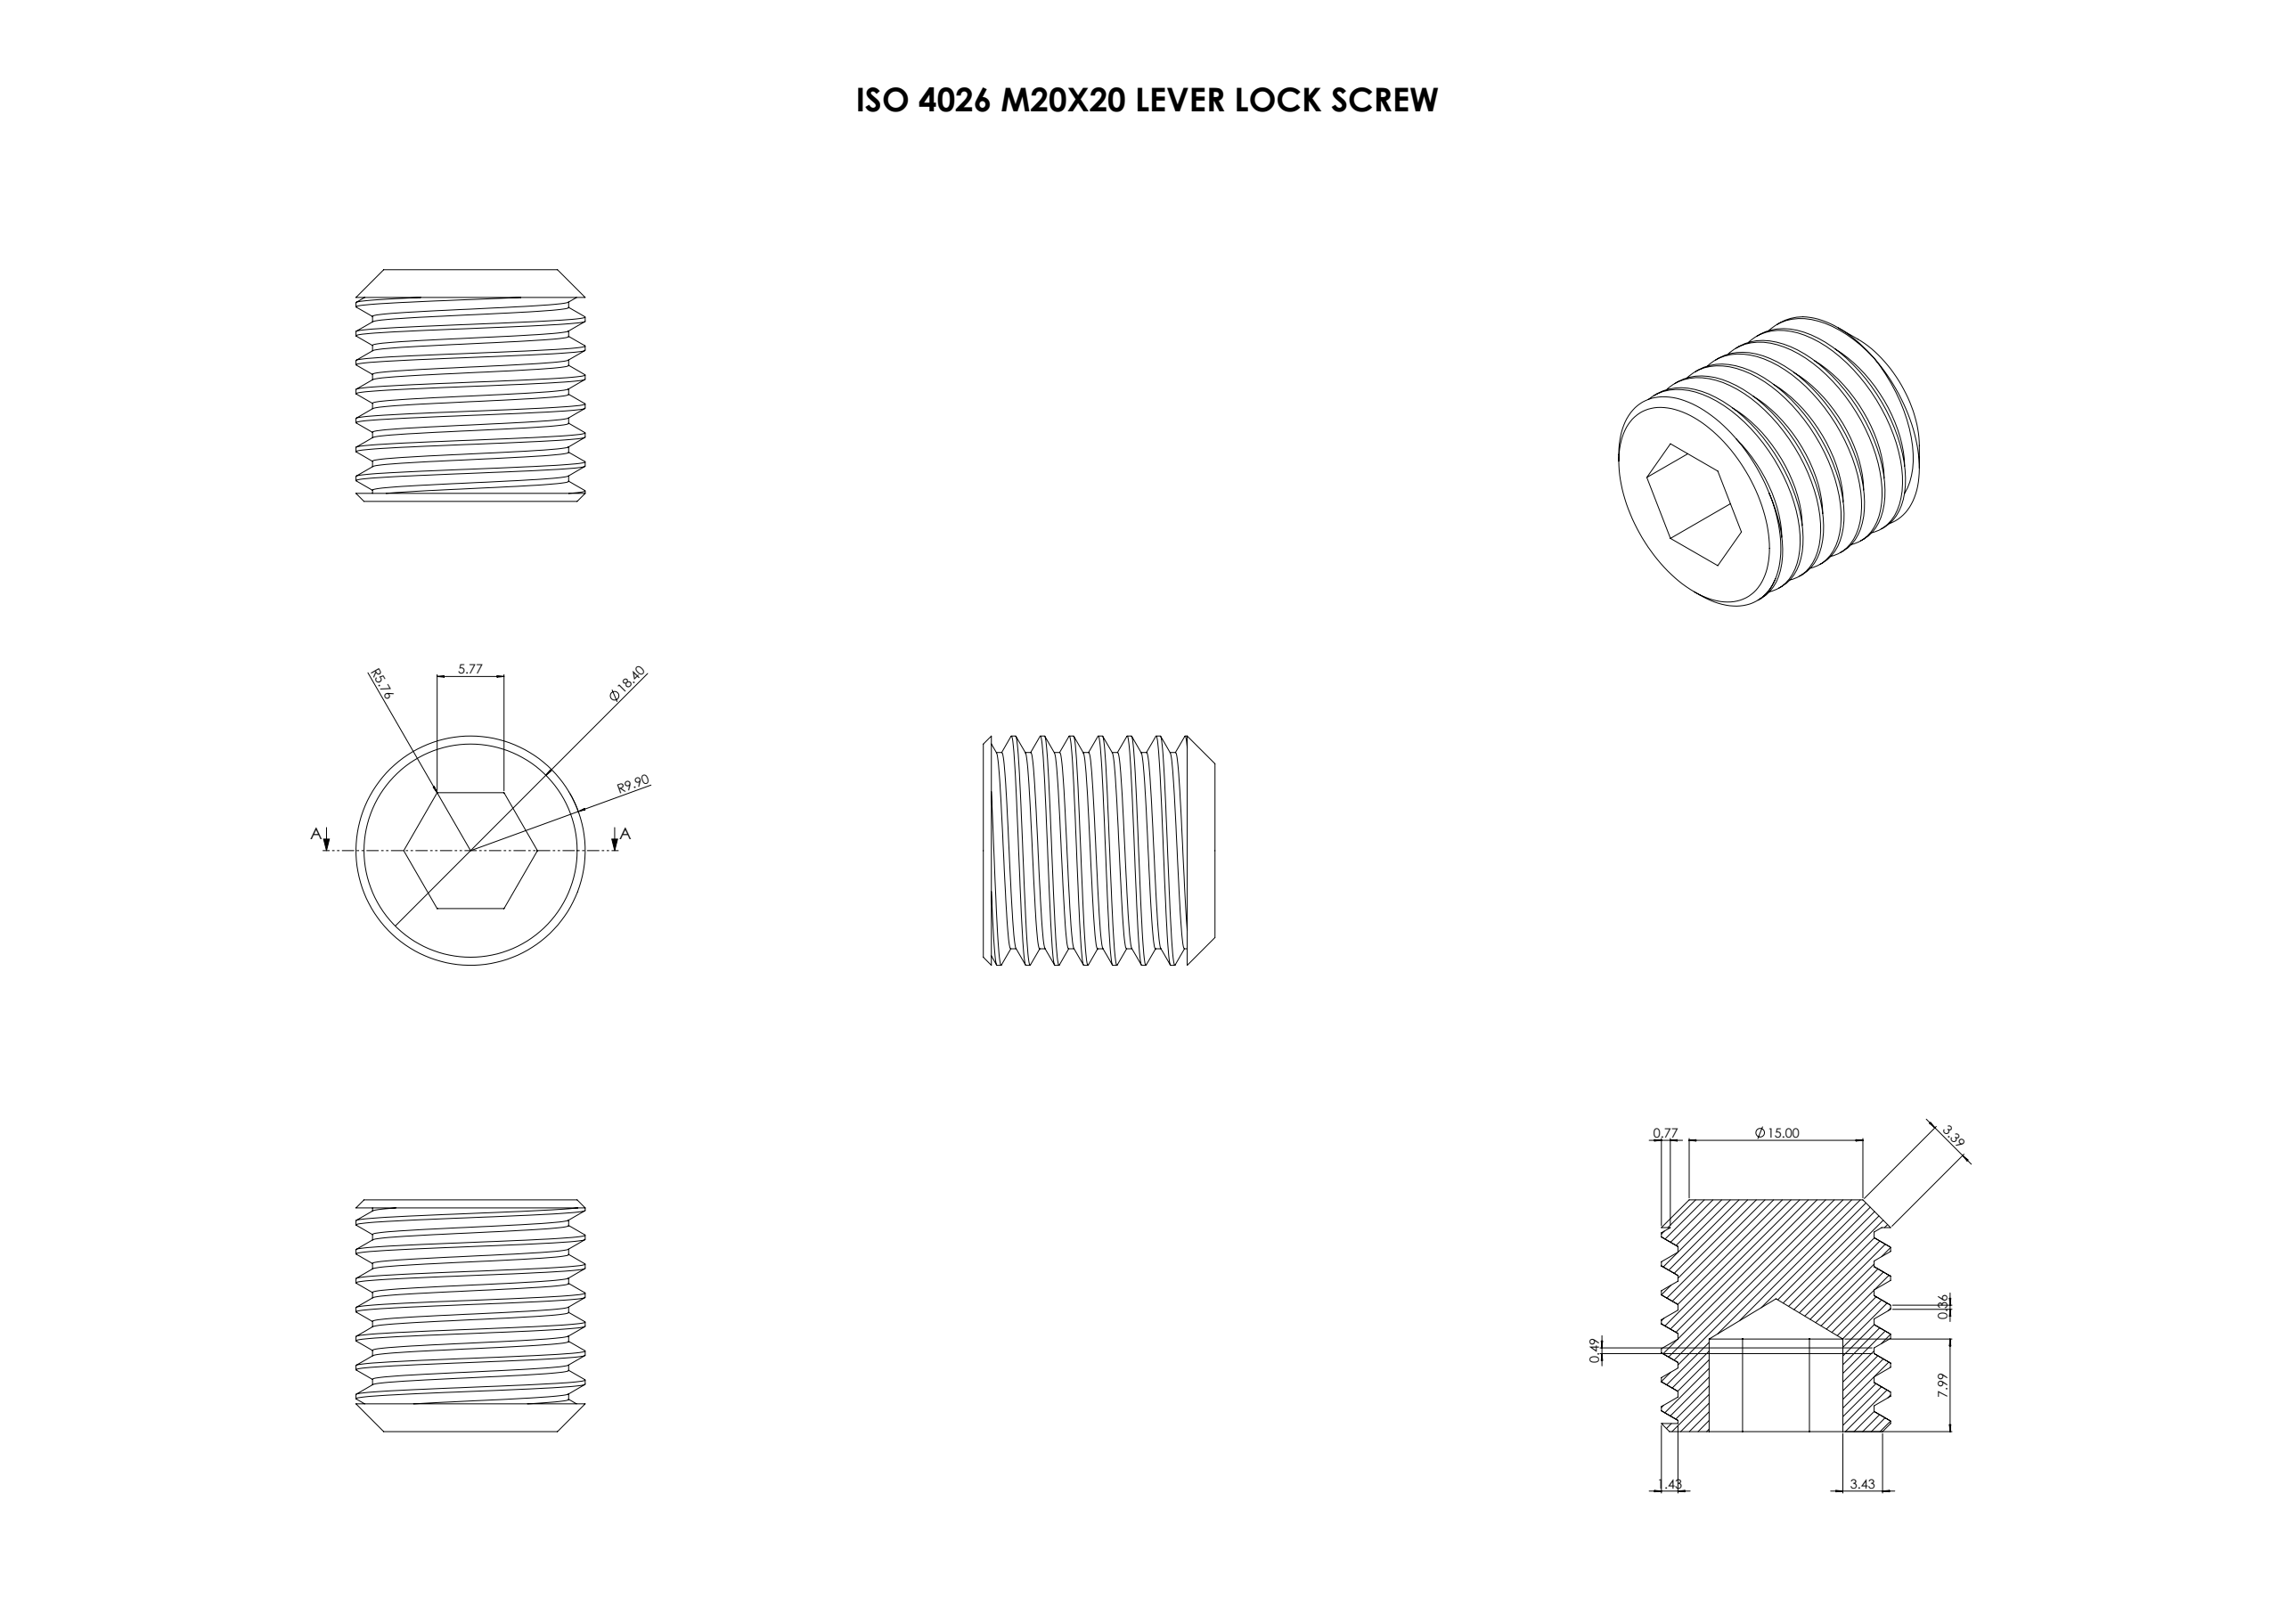
ISO-10303-21;
HEADER;
/* Generated by software containing ST-Developer
 * from STEP Tools, Inc. (www.steptools.com) 
 */

FILE_DESCRIPTION(
/* description */ (''),
/* implementation_level */ '2;1');

FILE_NAME(
/* name */ '15_ISO_4026_M20x20_Lever_Lock_Screw.step',
/* time_stamp */ '2026-10-19T23:58:09-07:00',
/* author */ (''),
/* organization */ (''),
/* preprocessor_version */ 'ST-DEVELOPER v20.2',
/* originating_system */ 'Autodesk Translation Framework v15.15.0.0',
/* authorisation */ '');

FILE_SCHEMA (('AP203_CONFIGURATION_CONTROLLED_3D_DESIGN_OF_MECHANICAL_PARTS_AND_ASSEMBLIES_MIM_LF { 1 0 10303 203 3 1 4 }',
'AUTOMOTIVE_DESIGN { 1 0 10303 214 3 1 1 }','INTEGRATED_CNC_SCHEMA','MODEL_BASED_INTEGRATED_MANUFACTURING_SCHEMA',
'PROCESS_PLANNING_SCHEMA','AP242_MANAGED_MODEL_BASED_3D_ENGINEERING_MIM_LF { 1 0 10303 442 3 1 4 }'));
ENDSEC;

DATA;
#10=MECHANICAL_DESIGN_GEOMETRIC_PRESENTATION_REPRESENTATION('',(#412),#70757);
#203=(
BOUNDED_CURVE()
B_SPLINE_CURVE(2,(#47308,#47309,#47310),.UNSPECIFIED.,.F.,.F.)
B_SPLINE_CURVE_WITH_KNOTS((3,3),(0.,0.00348481894602421),.UNSPECIFIED.)
CURVE()
GEOMETRIC_REPRESENTATION_ITEM()
RATIONAL_B_SPLINE_CURVE((1.,1.00000419109631,1.))
REPRESENTATION_ITEM('')
);
#204=(
BOUNDED_CURVE()
B_SPLINE_CURVE(2,(#47312,#47313,#47314),.UNSPECIFIED.,.F.,.F.)
B_SPLINE_CURVE_WITH_KNOTS((3,3),(0.,0.0034848189460241),.UNSPECIFIED.)
CURVE()
GEOMETRIC_REPRESENTATION_ITEM()
RATIONAL_B_SPLINE_CURVE((1.,1.00000419078036,1.))
REPRESENTATION_ITEM('')
);
#205=(
BOUNDED_CURVE()
B_SPLINE_CURVE(2,(#47317,#47318,#47319),.UNSPECIFIED.,.F.,.F.)
B_SPLINE_CURVE_WITH_KNOTS((3,3),(0.,0.00348481894602397),.UNSPECIFIED.)
CURVE()
GEOMETRIC_REPRESENTATION_ITEM()
RATIONAL_B_SPLINE_CURVE((1.,1.00000419109938,1.))
REPRESENTATION_ITEM('')
);
#206=(
BOUNDED_CURVE()
B_SPLINE_CURVE(2,(#47321,#47322,#47323),.UNSPECIFIED.,.F.,.F.)
B_SPLINE_CURVE_WITH_KNOTS((3,3),(0.,0.00348481894602389),.UNSPECIFIED.)
CURVE()
GEOMETRIC_REPRESENTATION_ITEM()
RATIONAL_B_SPLINE_CURVE((1.,1.0000041910806,1.))
REPRESENTATION_ITEM('')
);
#207=(
BOUNDED_CURVE()
B_SPLINE_CURVE(2,(#47326,#47327,#47328),.UNSPECIFIED.,.F.,.F.)
B_SPLINE_CURVE_WITH_KNOTS((3,3),(0.,0.003484818946024),.UNSPECIFIED.)
CURVE()
GEOMETRIC_REPRESENTATION_ITEM()
RATIONAL_B_SPLINE_CURVE((1.,1.00000419096159,1.))
REPRESENTATION_ITEM('')
);
#208=(
BOUNDED_CURVE()
B_SPLINE_CURVE(2,(#47330,#47331,#47332),.UNSPECIFIED.,.F.,.F.)
B_SPLINE_CURVE_WITH_KNOTS((3,3),(0.,0.00348481894602396),.UNSPECIFIED.)
CURVE()
GEOMETRIC_REPRESENTATION_ITEM()
RATIONAL_B_SPLINE_CURVE((1.,1.00000419112827,1.))
REPRESENTATION_ITEM('')
);
#209=(
BOUNDED_CURVE()
B_SPLINE_CURVE(2,(#47335,#47336,#47337),.UNSPECIFIED.,.F.,.F.)
B_SPLINE_CURVE_WITH_KNOTS((3,3),(0.,0.00348481894602387),.UNSPECIFIED.)
CURVE()
GEOMETRIC_REPRESENTATION_ITEM()
RATIONAL_B_SPLINE_CURVE((1.,1.00000419105483,1.))
REPRESENTATION_ITEM('')
);
#210=(
BOUNDED_CURVE()
B_SPLINE_CURVE(2,(#47339,#47340,#47341),.UNSPECIFIED.,.F.,.F.)
B_SPLINE_CURVE_WITH_KNOTS((3,3),(0.,0.00348481894602378),.UNSPECIFIED.)
CURVE()
GEOMETRIC_REPRESENTATION_ITEM()
RATIONAL_B_SPLINE_CURVE((1.,1.00000419099658,1.))
REPRESENTATION_ITEM('')
);
#211=(
BOUNDED_CURVE()
B_SPLINE_CURVE(2,(#47344,#47345,#47346),.UNSPECIFIED.,.F.,.F.)
B_SPLINE_CURVE_WITH_KNOTS((3,3),(0.,0.00348481894602419),.UNSPECIFIED.)
CURVE()
GEOMETRIC_REPRESENTATION_ITEM()
RATIONAL_B_SPLINE_CURVE((1.,1.00000419117121,1.))
REPRESENTATION_ITEM('')
);
#212=(
BOUNDED_CURVE()
B_SPLINE_CURVE(2,(#47348,#47349,#47350),.UNSPECIFIED.,.F.,.F.)
B_SPLINE_CURVE_WITH_KNOTS((3,3),(0.,0.00348481894602411),.UNSPECIFIED.)
CURVE()
GEOMETRIC_REPRESENTATION_ITEM()
RATIONAL_B_SPLINE_CURVE((1.,1.00000419088834,1.))
REPRESENTATION_ITEM('')
);
#213=(
BOUNDED_CURVE()
B_SPLINE_CURVE(2,(#47353,#47354,#47355),.UNSPECIFIED.,.F.,.F.)
B_SPLINE_CURVE_WITH_KNOTS((3,3),(0.,0.00348481894602378),.UNSPECIFIED.)
CURVE()
GEOMETRIC_REPRESENTATION_ITEM()
RATIONAL_B_SPLINE_CURVE((1.,1.00000419109063,1.))
REPRESENTATION_ITEM('')
);
#214=(
BOUNDED_CURVE()
B_SPLINE_CURVE(2,(#47357,#47358,#47359),.UNSPECIFIED.,.F.,.F.)
B_SPLINE_CURVE_WITH_KNOTS((3,3),(0.,0.00348481894602365),.UNSPECIFIED.)
CURVE()
GEOMETRIC_REPRESENTATION_ITEM()
RATIONAL_B_SPLINE_CURVE((1.,1.00000419111732,1.))
REPRESENTATION_ITEM('')
);
#274=B_SPLINE_SURFACE_WITH_KNOTS('',3,3,((#46301,#46302,#46303,#46304,#46305,
#46306,#46307,#46308,#46309,#46310,#46311,#46312,#46313,#46314,#46315,#46316,
#46317,#46318,#46319,#46320,#46321,#46322,#46323,#46324,#46325,#46326,#46327,
#46328,#46329,#46330,#46331,#46332,#46333,#46334,#46335,#46336,#46337,#46338,
#46339,#46340,#46341,#46342,#46343,#46344,#46345,#46346,#46347,#46348,#46349,
#46350,#46351,#46352,#46353,#46354,#46355,#46356,#46357,#46358,#46359,#46360,
#46361,#46362,#46363,#46364,#46365,#46366,#46367,#46368,#46369,#46370,#46371,
#46372,#46373,#46374,#46375,#46376,#46377,#46378,#46379,#46380,#46381,#46382,
#46383,#46384,#46385,#46386,#46387,#46388,#46389,#46390,#46391,#46392,#46393),
(#46394,#46395,#46396,#46397,#46398,#46399,#46400,#46401,#46402,#46403,
#46404,#46405,#46406,#46407,#46408,#46409,#46410,#46411,#46412,#46413,#46414,
#46415,#46416,#46417,#46418,#46419,#46420,#46421,#46422,#46423,#46424,#46425,
#46426,#46427,#46428,#46429,#46430,#46431,#46432,#46433,#46434,#46435,#46436,
#46437,#46438,#46439,#46440,#46441,#46442,#46443,#46444,#46445,#46446,#46447,
#46448,#46449,#46450,#46451,#46452,#46453,#46454,#46455,#46456,#46457,#46458,
#46459,#46460,#46461,#46462,#46463,#46464,#46465,#46466,#46467,#46468,#46469,
#46470,#46471,#46472,#46473,#46474,#46475,#46476,#46477,#46478,#46479,#46480,
#46481,#46482,#46483,#46484,#46485,#46486),(#46487,#46488,#46489,#46490,
#46491,#46492,#46493,#46494,#46495,#46496,#46497,#46498,#46499,#46500,#46501,
#46502,#46503,#46504,#46505,#46506,#46507,#46508,#46509,#46510,#46511,#46512,
#46513,#46514,#46515,#46516,#46517,#46518,#46519,#46520,#46521,#46522,#46523,
#46524,#46525,#46526,#46527,#46528,#46529,#46530,#46531,#46532,#46533,#46534,
#46535,#46536,#46537,#46538,#46539,#46540,#46541,#46542,#46543,#46544,#46545,
#46546,#46547,#46548,#46549,#46550,#46551,#46552,#46553,#46554,#46555,#46556,
#46557,#46558,#46559,#46560,#46561,#46562,#46563,#46564,#46565,#46566,#46567,
#46568,#46569,#46570,#46571,#46572,#46573,#46574,#46575,#46576,#46577,#46578,
#46579),(#46580,#46581,#46582,#46583,#46584,#46585,#46586,#46587,#46588,
#46589,#46590,#46591,#46592,#46593,#46594,#46595,#46596,#46597,#46598,#46599,
#46600,#46601,#46602,#46603,#46604,#46605,#46606,#46607,#46608,#46609,#46610,
#46611,#46612,#46613,#46614,#46615,#46616,#46617,#46618,#46619,#46620,#46621,
#46622,#46623,#46624,#46625,#46626,#46627,#46628,#46629,#46630,#46631,#46632,
#46633,#46634,#46635,#46636,#46637,#46638,#46639,#46640,#46641,#46642,#46643,
#46644,#46645,#46646,#46647,#46648,#46649,#46650,#46651,#46652,#46653,#46654,
#46655,#46656,#46657,#46658,#46659,#46660,#46661,#46662,#46663,#46664,#46665,
#46666,#46667,#46668,#46669,#46670,#46671,#46672)),.UNSPECIFIED.,.F.,.F.,
 .F.,(4,4),(4,1,1,1,1,1,1,1,1,1,1,1,1,1,1,1,1,1,1,1,1,1,1,1,1,1,1,1,1,1,
1,1,1,1,1,1,1,1,1,1,1,1,1,1,1,1,1,1,1,1,1,1,1,1,1,1,1,1,1,1,1,1,1,1,1,1,
1,1,1,1,1,1,1,1,1,1,1,1,1,1,1,1,1,1,1,1,1,1,1,1,4),(0.,0.164689164286341),
(8.30638927278254,8.80158653784135,9.29678380290015,9.79198106795896,10.2871783330178,
10.7823755980766,11.2775728631354,11.7727701281942,12.267967393253,12.7631646583118,
13.2583619233706,13.7535591884294,14.2487564534882,14.743953718547,15.2391509836058,
15.7343482486646,16.2295455137234,16.7247427787822,17.219940043841,17.7151373088998,
18.2103345739587,18.7055318390175,19.2007291040763,19.6959263691351,20.1911236341939,
20.6863208992527,21.1815181643115,21.6767154293703,22.1719126944291,22.6671099594879,
23.1623072245467,23.6575044896055,24.1527017546643,24.6478990197231,25.1430962847819,
25.6382935498407,26.1334908148995,26.6286880799584,27.1238853450172,27.619082610076,
28.1142798751348,28.6094771401936,29.1046744052524,29.5998716703112,30.09506893537,
30.5902662004288,31.0854634654876,31.5806607305464,32.0758579956052,32.571055260664,
33.0662525257228,33.5614497907816,34.0566470558404,34.5518443208992,35.0470415859581,
35.5422388510169,36.0374361160757,36.5326333811345,37.0278306461933,37.5230279112521,
38.0182251763109,38.5134224413697,39.0086197064285,39.5038169714873,39.9990142365461,
40.4942115016049,40.9894087666637,41.4846060317225,41.9798032967813,42.4750005618401,
42.9701978268989,43.4653950919578,43.9605923570166,44.4557896220754,44.9509868871342,
45.446184152193,45.9413814172518,46.4365786823106,46.9317759473694,47.4269732124282,
47.922170477487,48.4173677425458,48.9125650076046,49.4077622726634,49.9029595377222,
50.398156802781,50.8933540678398,51.3885513328986,51.8837485979574,52.3789458630163,
52.8741431280751),.UNSPECIFIED.);
#275=B_SPLINE_SURFACE_WITH_KNOTS('',3,3,((#46887,#46888,#46889,#46890,#46891,
#46892,#46893,#46894,#46895,#46896,#46897,#46898,#46899,#46900,#46901,#46902,
#46903,#46904,#46905,#46906,#46907,#46908,#46909,#46910,#46911,#46912,#46913,
#46914,#46915,#46916,#46917,#46918,#46919,#46920,#46921,#46922,#46923,#46924,
#46925,#46926,#46927,#46928,#46929,#46930,#46931,#46932,#46933,#46934,#46935,
#46936,#46937,#46938,#46939,#46940,#46941,#46942,#46943,#46944,#46945,#46946,
#46947,#46948,#46949,#46950,#46951,#46952,#46953,#46954,#46955,#46956,#46957,
#46958,#46959,#46960,#46961,#46962,#46963,#46964,#46965,#46966,#46967,#46968,
#46969,#46970,#46971,#46972,#46973,#46974,#46975,#46976,#46977,#46978,#46979),
(#46980,#46981,#46982,#46983,#46984,#46985,#46986,#46987,#46988,#46989,
#46990,#46991,#46992,#46993,#46994,#46995,#46996,#46997,#46998,#46999,#47000,
#47001,#47002,#47003,#47004,#47005,#47006,#47007,#47008,#47009,#47010,#47011,
#47012,#47013,#47014,#47015,#47016,#47017,#47018,#47019,#47020,#47021,#47022,
#47023,#47024,#47025,#47026,#47027,#47028,#47029,#47030,#47031,#47032,#47033,
#47034,#47035,#47036,#47037,#47038,#47039,#47040,#47041,#47042,#47043,#47044,
#47045,#47046,#47047,#47048,#47049,#47050,#47051,#47052,#47053,#47054,#47055,
#47056,#47057,#47058,#47059,#47060,#47061,#47062,#47063,#47064,#47065,#47066,
#47067,#47068,#47069,#47070,#47071,#47072),(#47073,#47074,#47075,#47076,
#47077,#47078,#47079,#47080,#47081,#47082,#47083,#47084,#47085,#47086,#47087,
#47088,#47089,#47090,#47091,#47092,#47093,#47094,#47095,#47096,#47097,#47098,
#47099,#47100,#47101,#47102,#47103,#47104,#47105,#47106,#47107,#47108,#47109,
#47110,#47111,#47112,#47113,#47114,#47115,#47116,#47117,#47118,#47119,#47120,
#47121,#47122,#47123,#47124,#47125,#47126,#47127,#47128,#47129,#47130,#47131,
#47132,#47133,#47134,#47135,#47136,#47137,#47138,#47139,#47140,#47141,#47142,
#47143,#47144,#47145,#47146,#47147,#47148,#47149,#47150,#47151,#47152,#47153,
#47154,#47155,#47156,#47157,#47158,#47159,#47160,#47161,#47162,#47163,#47164,
#47165),(#47166,#47167,#47168,#47169,#47170,#47171,#47172,#47173,#47174,
#47175,#47176,#47177,#47178,#47179,#47180,#47181,#47182,#47183,#47184,#47185,
#47186,#47187,#47188,#47189,#47190,#47191,#47192,#47193,#47194,#47195,#47196,
#47197,#47198,#47199,#47200,#47201,#47202,#47203,#47204,#47205,#47206,#47207,
#47208,#47209,#47210,#47211,#47212,#47213,#47214,#47215,#47216,#47217,#47218,
#47219,#47220,#47221,#47222,#47223,#47224,#47225,#47226,#47227,#47228,#47229,
#47230,#47231,#47232,#47233,#47234,#47235,#47236,#47237,#47238,#47239,#47240,
#47241,#47242,#47243,#47244,#47245,#47246,#47247,#47248,#47249,#47250,#47251,
#47252,#47253,#47254,#47255,#47256,#47257,#47258)),.UNSPECIFIED.,.F.,.F.,
 .F.,(4,4),(4,1,1,1,1,1,1,1,1,1,1,1,1,1,1,1,1,1,1,1,1,1,1,1,1,1,1,1,1,1,
1,1,1,1,1,1,1,1,1,1,1,1,1,1,1,1,1,1,1,1,1,1,1,1,1,1,1,1,1,1,1,1,1,1,1,1,
1,1,1,1,1,1,1,1,1,1,1,1,1,1,1,1,1,1,1,1,1,1,1,1,4),(0.,0.164689164286341),
(11.6152142277547,12.1104114928135,12.6056087578723,13.1008060229311,13.59600328799,
14.0912005530488,14.5863978181076,15.0815950831664,15.5767923482252,16.071989613284,
16.5671868783428,17.0623841434016,17.5575814084604,18.0527786735192,18.547975938578,
19.0431732036368,19.5383704686956,20.0335677337544,20.5287649988132,21.023962263872,
21.5191595289308,22.0143567939897,22.5095540590485,23.0047513241073,23.4999485891661,
23.9951458542249,24.4903431192837,24.9855403843425,25.4807376494013,25.9759349144601,
26.4711321795189,26.9663294445777,27.4615267096365,27.9567239746953,28.4519212397541,
28.9471185048129,29.4423157698717,29.9375130349305,30.4327102999894,30.9279075650482,
31.423104830107,31.9183020951658,32.4134993602246,32.9086966252834,33.4038938903422,
33.899091155401,34.3942884204598,34.8894856855186,35.3846829505774,35.8798802156362,
36.375077480695,36.8702747457538,37.3654720108126,37.8606692758714,38.3558665409303,
38.8510638059891,39.3462610710479,39.8414583361067,40.3366556011655,40.8318528662243,
41.3270501312831,41.8222473963419,42.3174446614007,42.8126419264595,43.3078391915183,
43.8030364565771,44.2982337216359,44.7934309866947,45.2886282517535,45.7838255168123,
46.2790227818711,46.7742200469299,47.2694173119888,47.7646145770476,48.2598118421064,
48.7550091071652,49.250206372224,49.7454036372828,50.2406009023416,50.7357981674004,
51.2309954324592,51.726192697518,52.2213899625768,52.7165872276356,53.2117844926944,
53.7069817577532,54.202179022812,54.6973762878708,55.1925735529296,55.6877708179885,
56.1829680830473),.UNSPECIFIED.);
#382=SHAPE_REPRESENTATION_RELATIONSHIP('SRR','None',#70823,#397);
#397=ADVANCED_BREP_SHAPE_REPRESENTATION('',(#472),#70747);
#412=STYLED_ITEM('',(#71054),#472);
#472=MANIFOLD_SOLID_BREP('Set screw',#26877);
#606=CYLINDRICAL_SURFACE('',#27433,0.989525);
#607=CYLINDRICAL_SURFACE('',#27435,0.989525);
#608=CYLINDRICAL_SURFACE('',#27436,0.989525);
#609=CYLINDRICAL_SURFACE('',#27437,0.989525);
#610=CYLINDRICAL_SURFACE('',#27438,0.989525);
#611=CYLINDRICAL_SURFACE('',#27439,0.989525);
#612=CYLINDRICAL_SURFACE('',#27440,0.989525);
#613=CYLINDRICAL_SURFACE('',#27441,0.8469);
#614=CYLINDRICAL_SURFACE('',#27443,0.8469);
#615=CYLINDRICAL_SURFACE('',#27445,0.8469);
#616=CYLINDRICAL_SURFACE('',#27446,0.8469);
#617=CYLINDRICAL_SURFACE('',#27447,0.8469);
#618=CYLINDRICAL_SURFACE('',#27448,0.8469);
#619=CYLINDRICAL_SURFACE('',#27449,0.8469);
#620=CYLINDRICAL_SURFACE('',#27457,0.8469);
#621=CYLINDRICAL_SURFACE('',#27505,0.989525);
#861=FACE_BOUND('',#4381,.T.);
#1135=B_SPLINE_CURVE_WITH_KNOTS('',3,(#45348,#45349,#45350,#45351,#45352,
#45353,#45354,#45355,#45356,#45357,#45358,#45359,#45360,#45361,#45362,#45363),
 .UNSPECIFIED.,.F.,.F.,(4,3,3,3,3,4),(-4.09274904019422,-3.96157812047045,
-3.46638085541164,-2.97118359035283,-2.47598632529403,-2.06954507459125),
 .UNSPECIFIED.);
#1136=B_SPLINE_CURVE_WITH_KNOTS('',3,(#45366,#45367,#45368,#45369,#45370,
#45371,#45372,#45373,#45374,#45375),.UNSPECIFIED.,.F.,.F.,(4,3,3,4),(0.,
0.495197265058804,0.990394530117612,1.11838868798682),.UNSPECIFIED.);
#1137=B_SPLINE_CURVE_WITH_KNOTS('',3,(#45380,#45381,#45382,#45383,#45384,
#45385,#45386,#45387,#45388,#45389,#45390,#45391,#45392,#45393,#45394,#45395,
#45396,#45397,#45398,#45399,#45400,#45401,#45402,#45403,#45404,#45405,#45406,
#45407,#45408,#45409,#45410,#45411,#45412,#45413,#45414,#45415,#45416,#45417,
#45418,#45419),.UNSPECIFIED.,.F.,.F.,(4,3,3,3,3,3,3,3,3,3,3,3,3,4),(-10.3759343473738,
-9.90394530117612,-9.40874803611731,-8.91355077105851,-8.4183535059997,
-7.9231562409409,-7.42795897588209,-6.93276171082328,-6.43756444576448,
-5.94236718070567,-5.44716991564687,-4.95197265058806,-4.45677538552925,
-4.09274904019422),.UNSPECIFIED.);
#1138=B_SPLINE_CURVE_WITH_KNOTS('',3,(#45420,#45421,#45422,#45423,#45424,
#45425,#45426,#45427,#45428,#45429,#45430,#45431,#45432,#45433,#45434,#45435,
#45436,#45437,#45438,#45439,#45440,#45441,#45442,#45443,#45444,#45445,#45446,
#45447,#45448,#45449,#45450,#45451,#45452,#45453,#45454,#45455,#45456,#45457,
#45458,#45459),.UNSPECIFIED.,.F.,.F.,(4,3,3,3,3,3,3,3,3,3,3,3,3,4),(1.11838868798682,
1.48559179517642,1.98078906023522,2.47598632529403,2.97118359035284,3.46638085541164,
3.96157812047045,4.45677538552925,4.95197265058806,5.44716991564687,5.94236718070567,
6.43756444576448,6.93276171082328,7.4015739951664),.UNSPECIFIED.);
#1139=B_SPLINE_CURVE_WITH_KNOTS('',3,(#45464,#45465,#45466,#45467,#45468,
#45469,#45470,#45471,#45472,#45473,#45474,#45475,#45476,#45477,#45478,#45479,
#45480,#45481,#45482,#45483,#45484,#45485,#45486,#45487,#45488,#45489,#45490,
#45491,#45492,#45493,#45494,#45495,#45496,#45497,#45498,#45499,#45500,#45501,
#45502,#45503,#45504,#45505,#45506),.UNSPECIFIED.,.F.,.F.,(4,3,3,3,3,3,
3,3,3,3,3,3,3,3,4),(-16.6591196545534,-16.3415097469406,-15.8463124818818,
-15.351115216823,-14.8559179517642,-14.3607206867054,-13.8655234216466,
-13.3703261565878,-12.875128891529,-12.3799316264701,-11.8847343614113,
-11.3895370963525,-10.8943398312937,-10.3991425662349,-10.3759343473738),
 .UNSPECIFIED.);
#1140=B_SPLINE_CURVE_WITH_KNOTS('',3,(#45507,#45508,#45509,#45510,#45511,
#45512,#45513,#45514,#45515,#45516,#45517,#45518,#45519,#45520,#45521,#45522,
#45523,#45524,#45525,#45526,#45527,#45528,#45529,#45530,#45531,#45532,#45533,
#45534,#45535,#45536,#45537,#45538,#45539,#45540,#45541,#45542,#45543,#45544,
#45545,#45546,#45547,#45548,#45549),.UNSPECIFIED.,.F.,.F.,(4,3,3,3,3,3,
3,3,3,3,3,3,3,3,4),(7.4015739951664,7.42795897588209,7.92315624094089,8.4183535059997,
8.9135507710585,9.40874803611731,9.90394530117612,10.3991425662349,10.8943398312937,
11.3895370963525,11.8847343614113,12.3799316264701,12.875128891529,13.3703261565878,
13.684759302346),.UNSPECIFIED.);
#1141=B_SPLINE_CURVE_WITH_KNOTS('',3,(#45554,#45555,#45556,#45557,#45558,
#45559,#45560,#45561,#45562,#45563,#45564,#45565,#45566,#45567,#45568,#45569,
#45570,#45571,#45572,#45573,#45574,#45575,#45576,#45577,#45578,#45579,#45580,
#45581,#45582,#45583,#45584,#45585,#45586,#45587,#45588,#45589,#45590,#45591,
#45592,#45593,#45594,#45595,#45596),.UNSPECIFIED.,.F.,.F.,(4,3,3,3,3,3,
3,3,3,3,3,3,3,3,4),(-22.942304961733,-22.7790741927051,-22.2838769276463,
-21.7886796625875,-21.2934823975287,-20.7982851324699,-20.303087867411,
-19.8078906023522,-19.3126933372934,-18.8174960722346,-18.3222988071758,
-17.827101542117,-17.3319042770582,-16.8367070119994,-16.6591196545534),
 .UNSPECIFIED.);
#1142=B_SPLINE_CURVE_WITH_KNOTS('',3,(#45597,#45598,#45599,#45600,#45601,
#45602,#45603,#45604,#45605,#45606,#45607,#45608,#45609,#45610,#45611,#45612,
#45613,#45614,#45615,#45616,#45617,#45618,#45619,#45620,#45621,#45622,#45623,
#45624,#45625,#45626,#45627,#45628,#45629,#45630,#45631,#45632,#45633,#45634,
#45635,#45636,#45637,#45638,#45639),.UNSPECIFIED.,.F.,.F.,(4,3,3,3,3,3,
3,3,3,3,3,3,3,3,4),(13.684759302346,13.8655234216466,14.3607206867054,14.8559179517642,
15.351115216823,15.8463124818818,16.3415097469406,16.8367070119994,17.3319042770582,
17.827101542117,18.3222988071758,18.8174960722346,19.3126933372934,19.8078906023522,
19.9679446095256),.UNSPECIFIED.);
#1143=B_SPLINE_CURVE_WITH_KNOTS('',3,(#45644,#45645,#45646,#45647,#45648,
#45649,#45650,#45651,#45652,#45653,#45654,#45655,#45656,#45657,#45658,#45659,
#45660,#45661,#45662,#45663,#45664,#45665,#45666,#45667,#45668,#45669,#45670,
#45671,#45672,#45673,#45674,#45675,#45676,#45677,#45678,#45679,#45680,#45681,
#45682,#45683,#45684,#45685,#45686),.UNSPECIFIED.,.F.,.F.,(4,3,3,3,3,3,
3,3,3,3,3,3,3,3,4),(-29.2254902689126,-29.2166386384695,-28.7214413734107,
-28.2262441083519,-27.7310468432931,-27.2358495782343,-26.7406523131755,
-26.2454550481167,-25.7502577830579,-25.2550605179991,-24.7598632529403,
-24.2646659878815,-23.7694687228227,-23.2742714577639,-22.942304961733),
 .UNSPECIFIED.);
#1144=B_SPLINE_CURVE_WITH_KNOTS('',3,(#45687,#45688,#45689,#45690,#45691,
#45692,#45693,#45694,#45695,#45696,#45697,#45698,#45699,#45700,#45701,#45702,
#45703,#45704,#45705,#45706,#45707,#45708,#45709,#45710,#45711,#45712,#45713,
#45714,#45715,#45716,#45717,#45718,#45719,#45720,#45721,#45722,#45723,#45724,
#45725,#45726,#45727,#45728,#45729),.UNSPECIFIED.,.F.,.F.,(4,3,3,3,3,3,
3,3,3,3,3,3,3,3,4),(19.9679446095256,20.303087867411,20.7982851324698,21.2934823975286,
21.7886796625875,22.2838769276463,22.7790741927051,23.2742714577639,23.7694687228227,
24.2646659878815,24.7598632529403,25.2550605179991,25.7502577830579,26.2454550481167,
26.2511299167052),.UNSPECIFIED.);
#1145=B_SPLINE_CURVE_WITH_KNOTS('',3,(#45734,#45735,#45736,#45737,#45738,
#45739,#45740,#45741,#45742,#45743,#45744,#45745,#45746,#45747,#45748,#45749,
#45750,#45751,#45752,#45753,#45754,#45755,#45756,#45757,#45758,#45759,#45760,
#45761,#45762,#45763,#45764,#45765,#45766,#45767,#45768,#45769,#45770,#45771,
#45772,#45773),.UNSPECIFIED.,.F.,.F.,(4,3,3,3,3,3,3,3,3,3,3,3,3,4),(-35.5086755760922,
-35.1590058191752,-34.6638085541164,-34.1686112890576,-33.6734140239988,
-33.17821675894,-32.6830194938812,-32.1878222288224,-31.6926249637636,-31.1974276987048,
-30.702230433646,-30.2070331685872,-29.7118359035283,-29.2254902689126),
 .UNSPECIFIED.);
#1146=B_SPLINE_CURVE_WITH_KNOTS('',3,(#45774,#45775,#45776,#45777,#45778,
#45779,#45780,#45781,#45782,#45783,#45784,#45785,#45786,#45787,#45788,#45789,
#45790,#45791,#45792,#45793,#45794,#45795,#45796,#45797,#45798,#45799,#45800,
#45801,#45802,#45803,#45804,#45805,#45806,#45807,#45808,#45809,#45810,#45811,
#45812,#45813),.UNSPECIFIED.,.F.,.F.,(4,3,3,3,3,3,3,3,3,3,3,3,3,4),(26.2511299167052,
26.7406523131755,27.2358495782343,27.7310468432931,28.2262441083519,28.7214413734107,
29.2166386384696,29.7118359035284,30.2070331685872,30.702230433646,31.1974276987048,
31.6926249637636,32.1878222288224,32.5343152238847),.UNSPECIFIED.);
#1147=B_SPLINE_CURVE_WITH_KNOTS('',3,(#45818,#45819,#45820,#45821,#45822,
#45823,#45824,#45825,#45826,#45827,#45828,#45829,#45830,#45831,#45832,#45833,
#45834,#45835,#45836,#45837,#45838,#45839,#45840,#45841,#45842,#45843,#45844,
#45845,#45846,#45847,#45848,#45849,#45850,#45851,#45852,#45853,#45854,#45855,
#45856,#45857,#45858,#45859,#45860),.UNSPECIFIED.,.F.,.F.,(4,3,3,3,3,3,
3,3,3,3,3,3,3,3,4),(-41.7918608832718,-41.5965702649397,-41.1013729998809,
-40.6061757348221,-40.1109784697633,-39.6157812047045,-39.1205839396457,
-38.6253866745869,-38.1301894095281,-37.6349921444693,-37.1397948794104,
-36.6445976143516,-36.1494003492928,-35.654203084234,-35.5086755760922),
 .UNSPECIFIED.);
#1148=B_SPLINE_CURVE_WITH_KNOTS('',3,(#45861,#45862,#45863,#45864,#45865,
#45866,#45867,#45868,#45869,#45870,#45871,#45872,#45873,#45874,#45875,#45876,
#45877,#45878,#45879,#45880,#45881,#45882,#45883,#45884,#45885,#45886,#45887,
#45888,#45889,#45890,#45891,#45892,#45893,#45894,#45895,#45896,#45897,#45898,
#45899,#45900,#45901,#45902,#45903),.UNSPECIFIED.,.F.,.F.,(4,3,3,3,3,3,
3,3,3,3,3,3,3,3,4),(32.5343152238847,32.6830194938812,33.17821675894,33.6734140239988,
34.1686112890576,34.6638085541164,35.1590058191752,35.654203084234,36.1494003492928,
36.6445976143516,37.1397948794104,37.6349921444692,38.130189409528,38.6253866745868,
38.8175005310643),.UNSPECIFIED.);
#1149=B_SPLINE_CURVE_WITH_KNOTS('',3,(#45909,#45910,#45911,#45912,#45913),
 .UNSPECIFIED.,.F.,.F.,(4,1,4),(53.4070751110265,53.7069817577532,54.113423008456),
 .UNSPECIFIED.);
#1150=B_SPLINE_CURVE_WITH_KNOTS('',3,(#45919,#45920,#45921,#45922,#45923,
#45924,#45925,#45926,#45927,#45928,#45929,#45930,#45931,#45932,#45933,#45934,
#45935),.UNSPECIFIED.,.F.,.F.,(4,1,1,1,1,1,1,1,1,1,1,1,1,1,4),(47.1238898038469,
47.2694173119888,47.7646145770476,48.2598118421064,48.7550091071652,49.250206372224,
49.7454036372828,50.2406009023416,50.7357981674004,51.2309954324592,51.726192697518,
52.2213899625768,52.7165872276356,53.2117844926944,53.4070751110265),
 .UNSPECIFIED.);
#1151=B_SPLINE_CURVE_WITH_KNOTS('',3,(#45938,#45939,#45940,#45941,#45942,
#45943,#45944,#45945,#45946,#45947,#45948,#45949,#45950,#45951,#45952),
 .UNSPECIFIED.,.F.,.F.,(4,1,1,1,1,1,1,1,1,1,1,1,4),(47.1238898038469,47.4269732124282,
47.922170477487,48.4173677425458,48.9125650076046,49.4077622726634,49.9029595377222,
50.398156802781,50.8933540678398,51.3885513328986,51.8837485979574,52.3789458630163,
52.8741431280751),.UNSPECIFIED.);
#1152=B_SPLINE_CURVE_WITH_KNOTS('',3,(#45957,#45958,#45959,#45960,#45961,
#45962,#45963,#45964,#45965,#45966,#45967,#45968,#45969,#45970,#45971,#45972),
 .UNSPECIFIED.,.F.,.F.,(4,1,1,1,1,1,1,1,1,1,1,1,1,4),(40.8407044966673,
41.3270501312831,41.8222473963419,42.3174446614007,42.8126419264595,43.3078391915183,
43.8030364565771,44.2982337216359,44.7934309866947,45.2886282517535,45.7838255168123,
46.2790227818711,46.7742200469299,47.1238898038469),.UNSPECIFIED.);
#1153=B_SPLINE_CURVE_WITH_KNOTS('',3,(#45973,#45974,#45975,#45976,#45977,
#45978,#45979,#45980,#45981,#45982,#45983,#45984,#45985,#45986,#45987,#45988,
#45989),.UNSPECIFIED.,.F.,.F.,(4,1,1,1,1,1,1,1,1,1,1,1,1,1,4),(40.8407044966673,
40.9894087666637,41.4846060317225,41.9798032967813,42.4750005618401,42.9701978268989,
43.4653950919578,43.9605923570166,44.4557896220754,44.9509868871342,45.446184152193,
45.9413814172518,46.4365786823106,46.9317759473694,47.1238898038469),
 .UNSPECIFIED.);
#1154=B_SPLINE_CURVE_WITH_KNOTS('',3,(#45994,#45995,#45996,#45997,#45998,
#45999,#46000,#46001,#46002,#46003,#46004,#46005,#46006,#46007,#46008,#46009,
#46010),.UNSPECIFIED.,.F.,.F.,(4,1,1,1,1,1,1,1,1,1,1,1,1,1,4),(34.5575191894877,
34.8894856855186,35.3846829505774,35.8798802156362,36.375077480695,36.8702747457538,
37.3654720108126,37.8606692758714,38.3558665409303,38.8510638059891,39.3462610710479,
39.8414583361067,40.3366556011655,40.8318528662243,40.8407044966673),
 .UNSPECIFIED.);
#1155=B_SPLINE_CURVE_WITH_KNOTS('',3,(#46011,#46012,#46013,#46014,#46015,
#46016,#46017,#46018,#46019,#46020,#46021,#46022,#46023,#46024,#46025,#46026),
 .UNSPECIFIED.,.F.,.F.,(4,1,1,1,1,1,1,1,1,1,1,1,1,4),(34.5575191894877,
35.0470415859581,35.5422388510169,36.0374361160757,36.5326333811345,37.0278306461933,
37.5230279112521,38.0182251763109,38.5134224413697,39.0086197064285,39.5038169714873,
39.9990142365461,40.4942115016049,40.8407044966673),.UNSPECIFIED.);
#1156=B_SPLINE_CURVE_WITH_KNOTS('',3,(#46031,#46032,#46033,#46034,#46035,
#46036,#46037,#46038,#46039,#46040,#46041,#46042,#46043,#46044,#46045,#46046,
#46047),.UNSPECIFIED.,.F.,.F.,(4,1,1,1,1,1,1,1,1,1,1,1,1,1,4),(28.2743338823081,
28.4519212397541,28.9471185048129,29.4423157698717,29.9375130349305,30.4327102999894,
30.9279075650482,31.423104830107,31.9183020951658,32.4134993602246,32.9086966252834,
33.4038938903422,33.899091155401,34.3942884204598,34.5575191894877),
 .UNSPECIFIED.);
#1157=B_SPLINE_CURVE_WITH_KNOTS('',3,(#46048,#46049,#46050,#46051,#46052,
#46053,#46054,#46055,#46056,#46057,#46058,#46059,#46060,#46061,#46062,#46063,
#46064),.UNSPECIFIED.,.F.,.F.,(4,1,1,1,1,1,1,1,1,1,1,1,1,1,4),(28.2743338823081,
28.6094771401936,29.1046744052524,29.5998716703112,30.09506893537,30.5902662004288,
31.0854634654876,31.5806607305464,32.0758579956052,32.571055260664,33.0662525257228,
33.5614497907816,34.0566470558404,34.5518443208992,34.5575191894877),
 .UNSPECIFIED.);
#1158=B_SPLINE_CURVE_WITH_KNOTS('',3,(#46069,#46070,#46071,#46072,#46073,
#46074,#46075,#46076,#46077,#46078,#46079,#46080,#46081,#46082,#46083,#46084,
#46085),.UNSPECIFIED.,.F.,.F.,(4,1,1,1,1,1,1,1,1,1,1,1,1,1,4),(21.9911485751285,
22.0143567939897,22.5095540590485,23.0047513241073,23.4999485891661,23.9951458542249,
24.4903431192837,24.9855403843425,25.4807376494013,25.9759349144601,26.4711321795189,
26.9663294445777,27.4615267096365,27.9567239746953,28.2743338823081),
 .UNSPECIFIED.);
#1159=B_SPLINE_CURVE_WITH_KNOTS('',3,(#46086,#46087,#46088,#46089,#46090,
#46091,#46092,#46093,#46094,#46095,#46096,#46097,#46098,#46099,#46100,#46101,
#46102),.UNSPECIFIED.,.F.,.F.,(4,1,1,1,1,1,1,1,1,1,1,1,1,1,4),(21.9911485751285,
22.1719126944291,22.6671099594879,23.1623072245467,23.6575044896055,24.1527017546643,
24.6478990197231,25.1430962847819,25.6382935498407,26.1334908148995,26.6286880799584,
27.1238853450172,27.619082610076,28.1142798751348,28.2743338823081),
 .UNSPECIFIED.);
#1160=B_SPLINE_CURVE_WITH_KNOTS('',3,(#46107,#46108,#46109,#46110,#46111,
#46112,#46113,#46114,#46115,#46116,#46117,#46118,#46119,#46120,#46121,#46122),
 .UNSPECIFIED.,.F.,.F.,(4,1,1,1,1,1,1,1,1,1,1,1,1,4),(15.7079632679489,
16.071989613284,16.5671868783428,17.0623841434016,17.5575814084604,18.0527786735192,
18.547975938578,19.0431732036368,19.5383704686956,20.0335677337544,20.5287649988132,
21.023962263872,21.5191595289308,21.9911485751285),.UNSPECIFIED.);
#1161=B_SPLINE_CURVE_WITH_KNOTS('',3,(#46123,#46124,#46125,#46126,#46127,
#46128,#46129,#46130,#46131,#46132,#46133,#46134,#46135,#46136,#46137,#46138,
#46139),.UNSPECIFIED.,.F.,.F.,(4,1,1,1,1,1,1,1,1,1,1,1,1,1,4),(15.7079632679489,
15.7343482486646,16.2295455137234,16.7247427787822,17.219940043841,17.7151373088998,
18.2103345739587,18.7055318390175,19.2007291040763,19.6959263691351,20.1911236341939,
20.6863208992527,21.1815181643115,21.6767154293703,21.9911485751285),
 .UNSPECIFIED.);
#1162=B_SPLINE_CURVE_WITH_KNOTS('',3,(#46142,#46143,#46144,#46145,#46146,
#46147,#46148,#46149,#46150,#46151,#46152,#46153,#46154,#46155,#46156,#46157,
#46158,#46159,#46160,#46161,#46162,#46163,#46164,#46165,#46166,#46167,#46168,
#46169,#46170,#46171,#46172,#46173,#46174,#46175,#46176,#46177,#46178,#46179,
#46180,#46181,#46182,#46183,#46184,#46185,#46186,#46187,#46188,#46189,#46190,
#46191,#46192,#46193,#46194,#46195,#46196,#46197,#46198,#46199,#46200,#46201,
#46202,#46203,#46204,#46205,#46206,#46207,#46208,#46209,#46210,#46211,#46212,
#46213,#46214,#46215,#46216,#46217),.UNSPECIFIED.,.F.,.F.,(4,3,3,3,3,3,
3,3,3,3,3,3,3,3,3,3,3,3,3,3,3,3,3,3,3,4),(-1.91386167632963,-1.83787666420088,
-1.72938395031299,-1.69638705507551,-1.66779038111967,-1.54802690914779,
-1.46245266964146,-1.43449001143917,-1.40390580864931,-1.28249728337303,
-1.19581509431375,-1.13105418444924,-1.10714354766822,-0.982416794980164,
-0.952469860823683,-0.835450486557249,-0.774018515207216,-0.748138511354911,
-0.616265437556429,-0.484392363757948,-0.423843318288204,-0.388665671195739,
-0.36353285337654,-0.234458855956312,-0.104218518256837,0.),
 .UNSPECIFIED.);
#1163=B_SPLINE_CURVE_WITH_KNOTS('',3,(#46222,#46223,#46224,#46225,#46226,
#46227,#46228,#46229,#46230,#46231,#46232,#46233,#46234,#46235,#46236,#46237,
#46238,#46239,#46240,#46241,#46242,#46243,#46244,#46245,#46246,#46247,#46248,
#46249,#46250,#46251,#46252,#46253,#46254,#46255,#46256,#46257,#46258,#46259,
#46260,#46261,#46262,#46263,#46264,#46265,#46266,#46267,#46268,#46269,#46270,
#46271,#46272,#46273,#46274,#46275,#46276,#46277,#46278,#46279,#46280,#46281,
#46282,#46283,#46284,#46285,#46286,#46287,#46288,#46289,#46290,#46291,#46292,
#46293,#46294,#46295,#46296,#46297,#46298,#46299,#46300),.UNSPECIFIED.,
 .F.,.F.,(4,3,3,3,3,3,3,3,3,3,3,3,3,3,3,3,3,3,3,3,3,3,3,3,3,3,4),(-1.90760546354383,
-1.81998897247625,-1.70019436157863,-1.65920884954384,-1.62916942004787,
-1.50064906159473,-1.41275923540419,-1.38440638426796,-1.34081052888579,
-1.21430756052813,-1.088913657374,-1.03595243864197,-1.0113746483739,-0.888053044233851,
-0.877312664850233,-0.765554368577898,-0.706871867177446,-0.68052011894822,
-0.656720355914381,-0.536198813546398,-0.430279479760896,-0.375078455320756,
-0.336309197496637,-0.311758984916726,-0.19334490167706,-0.0770967652264511,
0.),.UNSPECIFIED.);
#1164=B_SPLINE_CURVE_WITH_KNOTS('',3,(#46673,#46674,#46675,#46676,#46677,
#46678,#46679,#46680,#46681,#46682,#46683,#46684,#46685,#46686,#46687,#46688,
#46689,#46690,#46691,#46692,#46693,#46694,#46695,#46696,#46697),
 .UNSPECIFIED.,.F.,.F.,(4,3,3,3,3,3,3,3,4),(38.8175005310643,39.1205839396457,
39.6157812047045,40.1109784697633,40.6061757348221,41.1013729998809,41.5965702649397,
42.0917675299985,42.4982087807013),.UNSPECIFIED.);
#1165=B_SPLINE_CURVE_WITH_KNOTS('',3,(#46699,#46700,#46701,#46702,#46703,
#46704,#46705,#46706,#46707,#46708,#46709,#46710,#46711,#46712,#46713,#46714,
#46715,#46716,#46717,#46718,#46719,#46720,#46721,#46722,#46723,#46724,#46725,
#46726,#46727,#46728,#46729,#46730,#46731,#46732,#46733,#46734,#46735,#46736,
#46737,#46738,#46739,#46740,#46741,#46742,#46743,#46744,#46745,#46746,#46747,
#46748,#46749,#46750,#46751,#46752,#46753,#46754,#46755,#46756,#46757,#46758,
#46759,#46760,#46761,#46762,#46763,#46764,#46765,#46766,#46767,#46768,#46769,
#46770,#46771,#46772,#46773,#46774),.UNSPECIFIED.,.F.,.F.,(4,3,3,3,3,3,
3,3,3,3,3,3,3,3,3,3,3,3,3,3,3,3,3,3,3,4),(-1.91386167632967,-1.83787666420092,
-1.72938395031302,-1.69638705987941,-1.66779038861988,-1.54802692650689,
-1.46245267849424,-1.4344900129501,-1.40390580864934,-1.28249727261198,
-1.19581511826659,-1.13105421602521,-1.10714359156754,-0.982416836462222,
-0.952469860823725,-0.835450486557284,-0.774018545328602,-0.748138537086926,
-0.616265450422444,-0.484392363757962,-0.423843318288217,-0.388665667195217,
-0.363532849728275,-0.234458958092049,-0.104218565736301,0.),
 .UNSPECIFIED.);
#1166=B_SPLINE_CURVE_WITH_KNOTS('',3,(#46775,#46776,#46777,#46778,#46779,
#46780,#46781,#46782,#46783,#46784,#46785,#46786,#46787,#46788),
 .UNSPECIFIED.,.F.,.F.,(4,1,1,1,1,1,1,1,1,1,1,4),(10.3759343473738,10.7823755980766,
11.2775728631354,11.7727701281942,12.267967393253,12.7631646583118,13.2583619233706,
13.7535591884294,14.2487564534882,14.743953718547,15.2391509836058,15.7079632679489),
 .UNSPECIFIED.);
#1167=B_SPLINE_CURVE_WITH_KNOTS('',3,(#46794,#46795,#46796,#46797,#46798,
#46799,#46800,#46801,#46802,#46803,#46804,#46805,#46806,#46807,#46808,#46809,
#46810,#46811,#46812,#46813,#46814,#46815,#46816,#46817,#46818,#46819,#46820,
#46821,#46822,#46823,#46824,#46825,#46826,#46827,#46828,#46829,#46830,#46831,
#46832,#46833,#46834,#46835,#46836,#46837,#46838,#46839,#46840,#46841,#46842,
#46843,#46844,#46845,#46846,#46847,#46848,#46849,#46850,#46851,#46852,#46853,
#46854,#46855,#46856,#46857,#46858,#46859,#46860,#46861,#46862,#46863,#46864,
#46865,#46866,#46867,#46868,#46869,#46870,#46871,#46872),.UNSPECIFIED.,
 .F.,.F.,(4,3,3,3,3,3,3,3,3,3,3,3,3,3,3,3,3,3,3,3,3,3,3,3,3,3,4),(-1.90760546354381,
-1.81998897247621,-1.7001943615786,-1.65920884369368,-1.62916941167379,
-1.50064905344499,-1.412759230544,-1.38440638462706,-1.34081052888577,-1.21430757107678,
-1.08891372531773,-1.03595283676006,-1.01137473308098,-0.888053166855498,
-0.877312664850218,-0.765554368577884,-0.706871875281147,-0.680520127214094,
-0.656720353469998,-0.536198723300522,-0.430279479760884,-0.375078429667684,
-0.33630914297151,-0.311758975914638,-0.193344896342556,-0.0770969253539728,
0.),.UNSPECIFIED.);
#1168=B_SPLINE_CURVE_WITH_KNOTS('',3,(#46875,#46876,#46877,#46878,#46879,
#46880,#46881,#46882,#46883,#46884,#46885,#46886),.UNSPECIFIED.,.F.,.F.,
(4,1,1,1,1,1,1,1,1,4),(11.6152142277547,12.1104114928135,12.6056087578723,
13.1008060229311,13.59600328799,14.0912005530488,14.5863978181076,15.0815950831664,
15.5767923482252,15.7079632679489),.UNSPECIFIED.);
#1169=B_SPLINE_CURVE_WITH_KNOTS('',3,(#47259,#47260,#47261,#47262,#47263,
#47264,#47265,#47266,#47267,#47268,#47269,#47270,#47271,#47272,#47273,#47274,
#47275,#47276,#47277),.UNSPECIFIED.,.F.,.F.,(4,3,3,3,3,3,4),(-44.5677538552925,
-44.0725565902337,-43.5773593251749,-43.0821620601161,-42.5869647950573,
-42.0917675299985,-41.7918608832718),.UNSPECIFIED.);
#1765=PLANE('',#27450);
#1766=PLANE('',#27453);
#1767=PLANE('',#27458);
#1768=PLANE('',#27460);
#1769=PLANE('',#27462);
#1770=PLANE('',#27464);
#1771=PLANE('',#27466);
#1772=PLANE('',#27468);
#1773=PLANE('',#27478);
#1774=PLANE('',#27479);
#1775=PLANE('',#27480);
#1776=PLANE('',#27481);
#1777=PLANE('',#27482);
#1778=PLANE('',#27483);
#1779=PLANE('',#27484);
#1780=PLANE('',#27485);
#1781=PLANE('',#27486);
#1782=PLANE('',#27487);
#1783=PLANE('',#27488);
#1784=PLANE('',#27489);
#1785=PLANE('',#27490);
#1786=PLANE('',#27491);
#1787=PLANE('',#27492);
#1788=PLANE('',#27493);
#1789=PLANE('',#27494);
#1790=PLANE('',#27495);
#1791=PLANE('',#27496);
#1792=PLANE('',#27497);
#1793=PLANE('',#27498);
#1794=PLANE('',#27499);
#1795=PLANE('',#27500);
#1796=PLANE('',#27501);
#1797=PLANE('',#27502);
#1798=PLANE('',#27509);
#2821=FACE_OUTER_BOUND('',#4326,.T.);
#2822=FACE_OUTER_BOUND('',#4327,.T.);
#2823=FACE_OUTER_BOUND('',#4328,.T.);
#2824=FACE_OUTER_BOUND('',#4329,.T.);
#2825=FACE_OUTER_BOUND('',#4330,.T.);
#2826=FACE_OUTER_BOUND('',#4331,.T.);
#2827=FACE_OUTER_BOUND('',#4332,.T.);
#2828=FACE_OUTER_BOUND('',#4333,.T.);
#2829=FACE_OUTER_BOUND('',#4334,.T.);
#2830=FACE_OUTER_BOUND('',#4335,.T.);
#2831=FACE_OUTER_BOUND('',#4336,.T.);
#2832=FACE_OUTER_BOUND('',#4337,.T.);
#2833=FACE_OUTER_BOUND('',#4338,.T.);
#2834=FACE_OUTER_BOUND('',#4339,.T.);
#2835=FACE_OUTER_BOUND('',#4340,.T.);
#2836=FACE_OUTER_BOUND('',#4341,.T.);
#2837=FACE_OUTER_BOUND('',#4342,.T.);
#2838=FACE_OUTER_BOUND('',#4343,.T.);
#2839=FACE_OUTER_BOUND('',#4344,.T.);
#2840=FACE_OUTER_BOUND('',#4345,.T.);
#2841=FACE_OUTER_BOUND('',#4346,.T.);
#2842=FACE_OUTER_BOUND('',#4347,.T.);
#2843=FACE_OUTER_BOUND('',#4348,.T.);
#2844=FACE_OUTER_BOUND('',#4349,.T.);
#2845=FACE_OUTER_BOUND('',#4350,.T.);
#2846=FACE_OUTER_BOUND('',#4351,.T.);
#2847=FACE_OUTER_BOUND('',#4352,.T.);
#2848=FACE_OUTER_BOUND('',#4353,.T.);
#2849=FACE_OUTER_BOUND('',#4354,.T.);
#2850=FACE_OUTER_BOUND('',#4355,.T.);
#2851=FACE_OUTER_BOUND('',#4356,.T.);
#2852=FACE_OUTER_BOUND('',#4357,.T.);
#2853=FACE_OUTER_BOUND('',#4358,.T.);
#2854=FACE_OUTER_BOUND('',#4359,.T.);
#2855=FACE_OUTER_BOUND('',#4360,.T.);
#2856=FACE_OUTER_BOUND('',#4361,.T.);
#2857=FACE_OUTER_BOUND('',#4362,.T.);
#2858=FACE_OUTER_BOUND('',#4363,.T.);
#2859=FACE_OUTER_BOUND('',#4364,.T.);
#2860=FACE_OUTER_BOUND('',#4365,.T.);
#2861=FACE_OUTER_BOUND('',#4366,.T.);
#2862=FACE_OUTER_BOUND('',#4367,.T.);
#2863=FACE_OUTER_BOUND('',#4368,.T.);
#2864=FACE_OUTER_BOUND('',#4369,.T.);
#2865=FACE_OUTER_BOUND('',#4370,.T.);
#2866=FACE_OUTER_BOUND('',#4371,.T.);
#2867=FACE_OUTER_BOUND('',#4372,.T.);
#2868=FACE_OUTER_BOUND('',#4373,.T.);
#2869=FACE_OUTER_BOUND('',#4374,.T.);
#2870=FACE_OUTER_BOUND('',#4375,.T.);
#2871=FACE_OUTER_BOUND('',#4376,.T.);
#2872=FACE_OUTER_BOUND('',#4377,.T.);
#2873=FACE_OUTER_BOUND('',#4378,.T.);
#2874=FACE_OUTER_BOUND('',#4379,.T.);
#2875=FACE_OUTER_BOUND('',#4380,.T.);
#4326=EDGE_LOOP('',(#18890,#18891,#18892,#18893));
#4327=EDGE_LOOP('',(#18894,#18895,#18896,#18897));
#4328=EDGE_LOOP('',(#18898,#18899,#18900,#18901));
#4329=EDGE_LOOP('',(#18902,#18903,#18904,#18905));
#4330=EDGE_LOOP('',(#18906,#18907,#18908,#18909));
#4331=EDGE_LOOP('',(#18910,#18911,#18912,#18913));
#4332=EDGE_LOOP('',(#18914,#18915,#18916,#18917));
#4333=EDGE_LOOP('',(#18918,#18919,#18920));
#4334=EDGE_LOOP('',(#18921,#18922,#18923,#18924,#18925));
#4335=EDGE_LOOP('',(#18926,#18927,#18928,#18929));
#4336=EDGE_LOOP('',(#18930,#18931,#18932,#18933));
#4337=EDGE_LOOP('',(#18934,#18935,#18936,#18937));
#4338=EDGE_LOOP('',(#18938,#18939,#18940,#18941));
#4339=EDGE_LOOP('',(#18942,#18943,#18944,#18945));
#4340=EDGE_LOOP('',(#18946,#18947,#18948,#18949,#18950,#18951));
#4341=EDGE_LOOP('',(#18952,#18953,#18954,#18955,#18956,#18957,#18958,#18959,
#18960,#18961,#18962,#18963,#18964,#18965,#18966,#18967,#18968));
#4342=EDGE_LOOP('',(#18969,#18970,#18971,#18972,#18973));
#4343=EDGE_LOOP('',(#18974,#18975,#18976,#18977));
#4344=EDGE_LOOP('',(#18978,#18979,#18980,#18981,#18982,#18983,#18984,#18985,
#18986,#18987,#18988,#18989,#18990,#18991,#18992,#18993,#18994,#18995));
#4345=EDGE_LOOP('',(#18996,#18997));
#4346=EDGE_LOOP('',(#18998,#18999));
#4347=EDGE_LOOP('',(#19000,#19001));
#4348=EDGE_LOOP('',(#19002,#19003));
#4349=EDGE_LOOP('',(#19004,#19005));
#4350=EDGE_LOOP('',(#19006,#19007));
#4351=EDGE_LOOP('',(#19008,#19009,#19010,#19011,#19012,#19013,#19014,#19015,
#19016,#19017,#19018,#19019,#19020,#19021,#19022,#19023,#19024,#19025,#19026,
#19027,#19028,#19029,#19030,#19031,#19032,#19033,#19034));
#4352=EDGE_LOOP('',(#19035,#19036,#19037,#19038));
#4353=EDGE_LOOP('',(#19039,#19040,#19041));
#4354=EDGE_LOOP('',(#19042,#19043,#19044,#19045));
#4355=EDGE_LOOP('',(#19046,#19047,#19048));
#4356=EDGE_LOOP('',(#19049,#19050,#19051));
#4357=EDGE_LOOP('',(#19052,#19053,#19054,#19055));
#4358=EDGE_LOOP('',(#19056,#19057,#19058));
#4359=EDGE_LOOP('',(#19059,#19060,#19061,#19062));
#4360=EDGE_LOOP('',(#19063,#19064,#19065));
#4361=EDGE_LOOP('',(#19066,#19067,#19068));
#4362=EDGE_LOOP('',(#19069,#19070,#19071));
#4363=EDGE_LOOP('',(#19072,#19073,#19074));
#4364=EDGE_LOOP('',(#19075,#19076,#19077));
#4365=EDGE_LOOP('',(#19078,#19079,#19080));
#4366=EDGE_LOOP('',(#19081,#19082,#19083));
#4367=EDGE_LOOP('',(#19084,#19085,#19086,#19087));
#4368=EDGE_LOOP('',(#19088,#19089,#19090,#19091));
#4369=EDGE_LOOP('',(#19092,#19093,#19094));
#4370=EDGE_LOOP('',(#19095,#19096,#19097));
#4371=EDGE_LOOP('',(#19098,#19099,#19100));
#4372=EDGE_LOOP('',(#19101,#19102,#19103,#19104));
#4373=EDGE_LOOP('',(#19105,#19106,#19107));
#4374=EDGE_LOOP('',(#19108,#19109,#19110));
#4375=EDGE_LOOP('',(#19111,#19112,#19113));
#4376=EDGE_LOOP('',(#19114));
#4377=EDGE_LOOP('',(#19115,#19116,#19117,#19118,#19119,#19120));
#4378=EDGE_LOOP('',(#19121,#19122,#19123,#19124));
#4379=EDGE_LOOP('',(#19125,#19126,#19127,#19128,#19129,#19130));
#4380=EDGE_LOOP('',(#19131));
#4381=EDGE_LOOP('',(#19132,#19133,#19134,#19135,#19136,#19137));
#5924=LINE('',#45346,#8421);
#5925=LINE('',#45379,#8422);
#5926=LINE('',#45463,#8423);
#5927=LINE('',#45553,#8424);
#5928=LINE('',#45643,#8425);
#5929=LINE('',#45733,#8426);
#5930=LINE('',#45817,#8427);
#5931=LINE('',#45907,#8428);
#5932=LINE('',#45918,#8429);
#5933=LINE('',#45956,#8430);
#5934=LINE('',#45993,#8431);
#5935=LINE('',#46030,#8432);
#5936=LINE('',#46068,#8433);
#5937=LINE('',#46106,#8434);
#5938=LINE('',#47281,#8435);
#5939=LINE('',#47285,#8436);
#5940=LINE('',#47289,#8437);
#5941=LINE('',#47293,#8438);
#5942=LINE('',#47297,#8439);
#5943=LINE('',#47300,#8440);
#5944=LINE('',#47305,#8441);
#5945=LINE('',#47363,#8442);
#5946=LINE('',#47365,#8443);
#5947=LINE('',#47366,#8444);
#5948=LINE('',#47369,#8445);
#5949=LINE('',#47370,#8446);
#5950=LINE('',#47373,#8447);
#5951=LINE('',#47374,#8448);
#5952=LINE('',#47377,#8449);
#5953=LINE('',#47378,#8450);
#5954=LINE('',#47381,#8451);
#5955=LINE('',#47382,#8452);
#5956=LINE('',#47385,#8453);
#5957=LINE('',#47386,#8454);
#5958=LINE('',#47389,#8455);
#5959=LINE('',#47390,#8456);
#5960=LINE('',#47393,#8457);
#5961=LINE('',#47394,#8458);
#5962=LINE('',#47397,#8459);
#5963=LINE('',#47398,#8460);
#5964=LINE('',#47400,#8461);
#5965=LINE('',#47402,#8462);
#5966=LINE('',#47405,#8463);
#5967=LINE('',#47408,#8464);
#5968=LINE('',#47409,#8465);
#5969=LINE('',#47411,#8466);
#5970=LINE('',#47413,#8467);
#5971=LINE('',#47416,#8468);
#5972=LINE('',#47417,#8469);
#5973=LINE('',#47419,#8470);
#5974=LINE('',#47423,#8471);
#5975=LINE('',#47431,#8472);
#5976=LINE('',#47437,#8473);
#8421=VECTOR('',#30041,1.);
#8422=VECTOR('',#30046,1.);
#8423=VECTOR('',#30049,1.);
#8424=VECTOR('',#30052,1.);
#8425=VECTOR('',#30055,1.);
#8426=VECTOR('',#30058,1.);
#8427=VECTOR('',#30061,1.);
#8428=VECTOR('',#30064,0.8469);
#8429=VECTOR('',#30069,0.8469);
#8430=VECTOR('',#30074,0.8469);
#8431=VECTOR('',#30077,0.8469);
#8432=VECTOR('',#30080,0.8469);
#8433=VECTOR('',#30083,0.8469);
#8434=VECTOR('',#30086,0.8469);
#8435=VECTOR('',#30105,1.);
#8436=VECTOR('',#30110,1.);
#8437=VECTOR('',#30115,1.);
#8438=VECTOR('',#30120,1.);
#8439=VECTOR('',#30125,1.);
#8440=VECTOR('',#30130,1.);
#8441=VECTOR('',#30135,0.288675134594813);
#8442=VECTOR('',#30152,1.);
#8443=VECTOR('',#30153,1.);
#8444=VECTOR('',#30154,1.);
#8445=VECTOR('',#30157,1.);
#8446=VECTOR('',#30158,1.);
#8447=VECTOR('',#30161,1.);
#8448=VECTOR('',#30162,1.);
#8449=VECTOR('',#30165,1.);
#8450=VECTOR('',#30166,1.);
#8451=VECTOR('',#30169,1.);
#8452=VECTOR('',#30170,1.);
#8453=VECTOR('',#30173,1.);
#8454=VECTOR('',#30174,1.);
#8455=VECTOR('',#30177,1.);
#8456=VECTOR('',#30178,1.);
#8457=VECTOR('',#30181,1.);
#8458=VECTOR('',#30182,1.);
#8459=VECTOR('',#30185,1.);
#8460=VECTOR('',#30186,1.);
#8461=VECTOR('',#30189,1.);
#8462=VECTOR('',#30192,1.);
#8463=VECTOR('',#30197,1.);
#8464=VECTOR('',#30200,1.);
#8465=VECTOR('',#30201,1.);
#8466=VECTOR('',#30204,1.);
#8467=VECTOR('',#30207,1.);
#8468=VECTOR('',#30210,1.);
#8469=VECTOR('',#30211,1.);
#8470=VECTOR('',#30214,1.);
#8471=VECTOR('',#30221,1.);
#8472=VECTOR('',#30234,0.875);
#8473=VECTOR('',#30243,0.96);
#10786=CIRCLE('',#27434,0.989525);
#10787=CIRCLE('',#27442,0.8469);
#10788=CIRCLE('',#27444,0.8469);
#10789=CIRCLE('',#27451,0.989525);
#10790=CIRCLE('',#27452,0.989525);
#10791=CIRCLE('',#27454,0.989525);
#10792=CIRCLE('',#27455,0.989525);
#10793=CIRCLE('',#27456,0.8469);
#10794=CIRCLE('',#27459,0.577350269189626);
#10795=CIRCLE('',#27461,0.577350269189626);
#10796=CIRCLE('',#27463,0.577350269189626);
#10797=CIRCLE('',#27465,0.577350269189626);
#10798=CIRCLE('',#27467,0.577350269189626);
#10799=CIRCLE('',#27469,0.577350269189626);
#10800=CIRCLE('',#27471,0.575688399926292);
#10801=CIRCLE('',#27472,0.575688399926292);
#10802=CIRCLE('',#27473,0.575688399926292);
#10803=CIRCLE('',#27474,0.575688399926292);
#10804=CIRCLE('',#27475,0.575688399926292);
#10805=CIRCLE('',#27476,0.575688399926292);
#10806=CIRCLE('',#27477,0.575688399926292);
#10807=CIRCLE('',#27503,0.75);
#10808=CIRCLE('',#27506,0.989525);
#10809=CIRCLE('',#27508,0.92);
#11592=VERTEX_POINT('',#45344);
#11593=VERTEX_POINT('',#45345);
#11594=VERTEX_POINT('',#45347);
#11595=VERTEX_POINT('',#45364);
#11596=VERTEX_POINT('',#45377);
#11597=VERTEX_POINT('',#45378);
#11598=VERTEX_POINT('',#45461);
#11599=VERTEX_POINT('',#45462);
#11600=VERTEX_POINT('',#45551);
#11601=VERTEX_POINT('',#45552);
#11602=VERTEX_POINT('',#45641);
#11603=VERTEX_POINT('',#45642);
#11604=VERTEX_POINT('',#45731);
#11605=VERTEX_POINT('',#45732);
#11606=VERTEX_POINT('',#45815);
#11607=VERTEX_POINT('',#45816);
#11608=VERTEX_POINT('',#45905);
#11609=VERTEX_POINT('',#45906);
#11610=VERTEX_POINT('',#45908);
#11611=VERTEX_POINT('',#45916);
#11612=VERTEX_POINT('',#45917);
#11613=VERTEX_POINT('',#45936);
#11614=VERTEX_POINT('',#45954);
#11615=VERTEX_POINT('',#45955);
#11616=VERTEX_POINT('',#45991);
#11617=VERTEX_POINT('',#45992);
#11618=VERTEX_POINT('',#46028);
#11619=VERTEX_POINT('',#46029);
#11620=VERTEX_POINT('',#46066);
#11621=VERTEX_POINT('',#46067);
#11622=VERTEX_POINT('',#46104);
#11623=VERTEX_POINT('',#46105);
#11624=VERTEX_POINT('',#46141);
#11625=VERTEX_POINT('',#46218);
#11626=VERTEX_POINT('',#46220);
#11627=VERTEX_POINT('',#46698);
#11628=VERTEX_POINT('',#46790);
#11629=VERTEX_POINT('',#46793);
#11630=VERTEX_POINT('',#47279);
#11631=VERTEX_POINT('',#47280);
#11632=VERTEX_POINT('',#47284);
#11633=VERTEX_POINT('',#47288);
#11634=VERTEX_POINT('',#47292);
#11635=VERTEX_POINT('',#47296);
#11636=VERTEX_POINT('',#47303);
#11637=VERTEX_POINT('',#47304);
#11638=VERTEX_POINT('',#47306);
#11639=VERTEX_POINT('',#47311);
#11640=VERTEX_POINT('',#47315);
#11641=VERTEX_POINT('',#47320);
#11642=VERTEX_POINT('',#47324);
#11643=VERTEX_POINT('',#47329);
#11644=VERTEX_POINT('',#47333);
#11645=VERTEX_POINT('',#47338);
#11646=VERTEX_POINT('',#47342);
#11647=VERTEX_POINT('',#47347);
#11648=VERTEX_POINT('',#47351);
#11649=VERTEX_POINT('',#47356);
#11650=VERTEX_POINT('',#47362);
#11651=VERTEX_POINT('',#47364);
#11652=VERTEX_POINT('',#47368);
#11653=VERTEX_POINT('',#47372);
#11654=VERTEX_POINT('',#47376);
#11655=VERTEX_POINT('',#47380);
#11656=VERTEX_POINT('',#47384);
#11657=VERTEX_POINT('',#47388);
#11658=VERTEX_POINT('',#47392);
#11659=VERTEX_POINT('',#47396);
#11660=VERTEX_POINT('',#47407);
#11661=VERTEX_POINT('',#47415);
#11662=VERTEX_POINT('',#47428);
#11663=VERTEX_POINT('',#47435);
#14298=EDGE_CURVE('',#11592,#11593,#5924,.T.);
#14299=EDGE_CURVE('',#11592,#11594,#1135,.T.);
#14300=EDGE_CURVE('',#11594,#11595,#10786,.T.);
#14301=EDGE_CURVE('',#11595,#11593,#1136,.T.);
#14302=EDGE_CURVE('',#11596,#11597,#5925,.T.);
#14303=EDGE_CURVE('',#11596,#11592,#1137,.T.);
#14304=EDGE_CURVE('',#11593,#11597,#1138,.T.);
#14305=EDGE_CURVE('',#11598,#11599,#5926,.T.);
#14306=EDGE_CURVE('',#11598,#11596,#1139,.T.);
#14307=EDGE_CURVE('',#11597,#11599,#1140,.T.);
#14308=EDGE_CURVE('',#11600,#11601,#5927,.T.);
#14309=EDGE_CURVE('',#11600,#11598,#1141,.T.);
#14310=EDGE_CURVE('',#11599,#11601,#1142,.T.);
#14311=EDGE_CURVE('',#11602,#11603,#5928,.T.);
#14312=EDGE_CURVE('',#11602,#11600,#1143,.T.);
#14313=EDGE_CURVE('',#11601,#11603,#1144,.T.);
#14314=EDGE_CURVE('',#11604,#11605,#5929,.T.);
#14315=EDGE_CURVE('',#11604,#11602,#1145,.T.);
#14316=EDGE_CURVE('',#11603,#11605,#1146,.T.);
#14317=EDGE_CURVE('',#11606,#11607,#5930,.T.);
#14318=EDGE_CURVE('',#11606,#11604,#1147,.T.);
#14319=EDGE_CURVE('',#11605,#11607,#1148,.T.);
#14320=EDGE_CURVE('',#11608,#11609,#5931,.T.);
#14321=EDGE_CURVE('',#11608,#11610,#1149,.T.);
#14322=EDGE_CURVE('',#11609,#11610,#10787,.T.);
#14323=EDGE_CURVE('',#11611,#11612,#5932,.T.);
#14324=EDGE_CURVE('',#11611,#11608,#1150,.T.);
#14325=EDGE_CURVE('',#11613,#11609,#10788,.T.);
#14326=EDGE_CURVE('',#11612,#11613,#1151,.T.);
#14327=EDGE_CURVE('',#11614,#11615,#5933,.T.);
#14328=EDGE_CURVE('',#11614,#11611,#1152,.T.);
#14329=EDGE_CURVE('',#11615,#11612,#1153,.T.);
#14330=EDGE_CURVE('',#11616,#11617,#5934,.T.);
#14331=EDGE_CURVE('',#11616,#11614,#1154,.T.);
#14332=EDGE_CURVE('',#11617,#11615,#1155,.T.);
#14333=EDGE_CURVE('',#11618,#11619,#5935,.T.);
#14334=EDGE_CURVE('',#11618,#11616,#1156,.T.);
#14335=EDGE_CURVE('',#11619,#11617,#1157,.T.);
#14336=EDGE_CURVE('',#11620,#11621,#5936,.T.);
#14337=EDGE_CURVE('',#11620,#11618,#1158,.T.);
#14338=EDGE_CURVE('',#11621,#11619,#1159,.T.);
#14339=EDGE_CURVE('',#11622,#11623,#5937,.T.);
#14340=EDGE_CURVE('',#11622,#11620,#1160,.T.);
#14341=EDGE_CURVE('',#11623,#11621,#1161,.T.);
#14342=EDGE_CURVE('',#11610,#11624,#1162,.T.);
#14343=EDGE_CURVE('',#11625,#11624,#10789,.F.);
#14344=EDGE_CURVE('',#11626,#11625,#10790,.F.);
#14345=EDGE_CURVE('',#11626,#11613,#1163,.T.);
#14346=EDGE_CURVE('',#11607,#11626,#1164,.T.);
#14347=EDGE_CURVE('',#11627,#11595,#1165,.T.);
#14348=EDGE_CURVE('',#11627,#11623,#1166,.T.);
#14349=EDGE_CURVE('',#11595,#11628,#10791,.T.);
#14350=EDGE_CURVE('',#11628,#11594,#10792,.T.);
#14351=EDGE_CURVE('',#11594,#11629,#1167,.T.);
#14352=EDGE_CURVE('',#11629,#11627,#10793,.T.);
#14353=EDGE_CURVE('',#11629,#11622,#1168,.T.);
#14354=EDGE_CURVE('',#11624,#11606,#1169,.T.);
#14355=EDGE_CURVE('',#11630,#11631,#5938,.T.);
#14356=EDGE_CURVE('',#11631,#11630,#10794,.T.);
#14357=EDGE_CURVE('',#11631,#11632,#5939,.T.);
#14358=EDGE_CURVE('',#11632,#11631,#10795,.T.);
#14359=EDGE_CURVE('',#11632,#11633,#5940,.T.);
#14360=EDGE_CURVE('',#11633,#11632,#10796,.T.);
#14361=EDGE_CURVE('',#11633,#11634,#5941,.T.);
#14362=EDGE_CURVE('',#11634,#11633,#10797,.T.);
#14363=EDGE_CURVE('',#11634,#11635,#5942,.T.);
#14364=EDGE_CURVE('',#11635,#11634,#10798,.T.);
#14365=EDGE_CURVE('',#11635,#11630,#5943,.T.);
#14366=EDGE_CURVE('',#11630,#11635,#10799,.T.);
#14367=EDGE_CURVE('',#11636,#11637,#5944,.T.);
#14368=EDGE_CURVE('',#11638,#11637,#10800,.T.);
#14369=EDGE_CURVE('',#11632,#11638,#203,.T.);
#14370=EDGE_CURVE('',#11639,#11631,#204,.T.);
#14371=EDGE_CURVE('',#11640,#11639,#10801,.T.);
#14372=EDGE_CURVE('',#11631,#11640,#205,.T.);
#14373=EDGE_CURVE('',#11641,#11630,#206,.T.);
#14374=EDGE_CURVE('',#11642,#11641,#10802,.T.);
#14375=EDGE_CURVE('',#11630,#11642,#207,.T.);
#14376=EDGE_CURVE('',#11643,#11635,#208,.T.);
#14377=EDGE_CURVE('',#11644,#11643,#10803,.T.);
#14378=EDGE_CURVE('',#11635,#11644,#209,.T.);
#14379=EDGE_CURVE('',#11645,#11634,#210,.T.);
#14380=EDGE_CURVE('',#11646,#11645,#10804,.T.);
#14381=EDGE_CURVE('',#11634,#11646,#211,.T.);
#14382=EDGE_CURVE('',#11647,#11633,#212,.T.);
#14383=EDGE_CURVE('',#11648,#11647,#10805,.T.);
#14384=EDGE_CURVE('',#11633,#11648,#213,.T.);
#14385=EDGE_CURVE('',#11649,#11632,#214,.T.);
#14386=EDGE_CURVE('',#11637,#11649,#10806,.T.);
#14387=EDGE_CURVE('',#11650,#11633,#5945,.T.);
#14388=EDGE_CURVE('',#11651,#11650,#5946,.T.);
#14389=EDGE_CURVE('',#11651,#11632,#5947,.T.);
#14390=EDGE_CURVE('',#11632,#11652,#5948,.T.);
#14391=EDGE_CURVE('',#11652,#11649,#5949,.T.);
#14392=EDGE_CURVE('',#11653,#11634,#5950,.T.);
#14393=EDGE_CURVE('',#11650,#11653,#5951,.T.);
#14394=EDGE_CURVE('',#11646,#11654,#5952,.T.);
#14395=EDGE_CURVE('',#11634,#11654,#5953,.T.);
#14396=EDGE_CURVE('',#11633,#11655,#5954,.T.);
#14397=EDGE_CURVE('',#11655,#11647,#5955,.T.);
#14398=EDGE_CURVE('',#11656,#11651,#5956,.T.);
#14399=EDGE_CURVE('',#11656,#11631,#5957,.T.);
#14400=EDGE_CURVE('',#11631,#11657,#5958,.T.);
#14401=EDGE_CURVE('',#11657,#11639,#5959,.T.);
#14402=EDGE_CURVE('',#11658,#11635,#5960,.T.);
#14403=EDGE_CURVE('',#11653,#11658,#5961,.T.);
#14404=EDGE_CURVE('',#11644,#11659,#5962,.T.);
#14405=EDGE_CURVE('',#11635,#11659,#5963,.T.);
#14406=EDGE_CURVE('',#11654,#11645,#5964,.T.);
#14407=EDGE_CURVE('',#11648,#11655,#5965,.T.);
#14408=EDGE_CURVE('',#11659,#11643,#5966,.T.);
#14409=EDGE_CURVE('',#11660,#11641,#5967,.T.);
#14410=EDGE_CURVE('',#11642,#11660,#5968,.T.);
#14411=EDGE_CURVE('',#11640,#11657,#5969,.T.);
#14412=EDGE_CURVE('',#11638,#11652,#5970,.T.);
#14413=EDGE_CURVE('',#11661,#11630,#5971,.T.);
#14414=EDGE_CURVE('',#11658,#11661,#5972,.T.);
#14415=EDGE_CURVE('',#11630,#11660,#5973,.T.);
#14416=EDGE_CURVE('',#11661,#11656,#5974,.T.);
#14417=EDGE_CURVE('',#11662,#11662,#10807,.T.);
#14418=EDGE_CURVE('',#11628,#11662,#5975,.T.);
#14419=EDGE_CURVE('',#11624,#11626,#10808,.F.);
#14420=EDGE_CURVE('',#11663,#11663,#10809,.T.);
#14421=EDGE_CURVE('',#11663,#11625,#5976,.T.);
#18890=ORIENTED_EDGE('',*,*,#14298,.F.);
#18891=ORIENTED_EDGE('',*,*,#14299,.T.);
#18892=ORIENTED_EDGE('',*,*,#14300,.T.);
#18893=ORIENTED_EDGE('',*,*,#14301,.T.);
#18894=ORIENTED_EDGE('',*,*,#14302,.F.);
#18895=ORIENTED_EDGE('',*,*,#14303,.T.);
#18896=ORIENTED_EDGE('',*,*,#14298,.T.);
#18897=ORIENTED_EDGE('',*,*,#14304,.T.);
#18898=ORIENTED_EDGE('',*,*,#14305,.F.);
#18899=ORIENTED_EDGE('',*,*,#14306,.T.);
#18900=ORIENTED_EDGE('',*,*,#14302,.T.);
#18901=ORIENTED_EDGE('',*,*,#14307,.T.);
#18902=ORIENTED_EDGE('',*,*,#14308,.F.);
#18903=ORIENTED_EDGE('',*,*,#14309,.T.);
#18904=ORIENTED_EDGE('',*,*,#14305,.T.);
#18905=ORIENTED_EDGE('',*,*,#14310,.T.);
#18906=ORIENTED_EDGE('',*,*,#14311,.F.);
#18907=ORIENTED_EDGE('',*,*,#14312,.T.);
#18908=ORIENTED_EDGE('',*,*,#14308,.T.);
#18909=ORIENTED_EDGE('',*,*,#14313,.T.);
#18910=ORIENTED_EDGE('',*,*,#14314,.F.);
#18911=ORIENTED_EDGE('',*,*,#14315,.T.);
#18912=ORIENTED_EDGE('',*,*,#14311,.T.);
#18913=ORIENTED_EDGE('',*,*,#14316,.T.);
#18914=ORIENTED_EDGE('',*,*,#14317,.F.);
#18915=ORIENTED_EDGE('',*,*,#14318,.T.);
#18916=ORIENTED_EDGE('',*,*,#14314,.T.);
#18917=ORIENTED_EDGE('',*,*,#14319,.T.);
#18918=ORIENTED_EDGE('',*,*,#14320,.F.);
#18919=ORIENTED_EDGE('',*,*,#14321,.T.);
#18920=ORIENTED_EDGE('',*,*,#14322,.F.);
#18921=ORIENTED_EDGE('',*,*,#14323,.F.);
#18922=ORIENTED_EDGE('',*,*,#14324,.T.);
#18923=ORIENTED_EDGE('',*,*,#14320,.T.);
#18924=ORIENTED_EDGE('',*,*,#14325,.F.);
#18925=ORIENTED_EDGE('',*,*,#14326,.F.);
#18926=ORIENTED_EDGE('',*,*,#14327,.F.);
#18927=ORIENTED_EDGE('',*,*,#14328,.T.);
#18928=ORIENTED_EDGE('',*,*,#14323,.T.);
#18929=ORIENTED_EDGE('',*,*,#14329,.F.);
#18930=ORIENTED_EDGE('',*,*,#14330,.F.);
#18931=ORIENTED_EDGE('',*,*,#14331,.T.);
#18932=ORIENTED_EDGE('',*,*,#14327,.T.);
#18933=ORIENTED_EDGE('',*,*,#14332,.F.);
#18934=ORIENTED_EDGE('',*,*,#14333,.F.);
#18935=ORIENTED_EDGE('',*,*,#14334,.T.);
#18936=ORIENTED_EDGE('',*,*,#14330,.T.);
#18937=ORIENTED_EDGE('',*,*,#14335,.F.);
#18938=ORIENTED_EDGE('',*,*,#14336,.F.);
#18939=ORIENTED_EDGE('',*,*,#14337,.T.);
#18940=ORIENTED_EDGE('',*,*,#14333,.T.);
#18941=ORIENTED_EDGE('',*,*,#14338,.F.);
#18942=ORIENTED_EDGE('',*,*,#14339,.F.);
#18943=ORIENTED_EDGE('',*,*,#14340,.T.);
#18944=ORIENTED_EDGE('',*,*,#14336,.T.);
#18945=ORIENTED_EDGE('',*,*,#14341,.F.);
#18946=ORIENTED_EDGE('',*,*,#14325,.T.);
#18947=ORIENTED_EDGE('',*,*,#14322,.T.);
#18948=ORIENTED_EDGE('',*,*,#14342,.T.);
#18949=ORIENTED_EDGE('',*,*,#14343,.F.);
#18950=ORIENTED_EDGE('',*,*,#14344,.F.);
#18951=ORIENTED_EDGE('',*,*,#14345,.T.);
#18952=ORIENTED_EDGE('',*,*,#14345,.F.);
#18953=ORIENTED_EDGE('',*,*,#14346,.F.);
#18954=ORIENTED_EDGE('',*,*,#14319,.F.);
#18955=ORIENTED_EDGE('',*,*,#14316,.F.);
#18956=ORIENTED_EDGE('',*,*,#14313,.F.);
#18957=ORIENTED_EDGE('',*,*,#14310,.F.);
#18958=ORIENTED_EDGE('',*,*,#14307,.F.);
#18959=ORIENTED_EDGE('',*,*,#14304,.F.);
#18960=ORIENTED_EDGE('',*,*,#14301,.F.);
#18961=ORIENTED_EDGE('',*,*,#14347,.F.);
#18962=ORIENTED_EDGE('',*,*,#14348,.T.);
#18963=ORIENTED_EDGE('',*,*,#14341,.T.);
#18964=ORIENTED_EDGE('',*,*,#14338,.T.);
#18965=ORIENTED_EDGE('',*,*,#14335,.T.);
#18966=ORIENTED_EDGE('',*,*,#14332,.T.);
#18967=ORIENTED_EDGE('',*,*,#14329,.T.);
#18968=ORIENTED_EDGE('',*,*,#14326,.T.);
#18969=ORIENTED_EDGE('',*,*,#14349,.T.);
#18970=ORIENTED_EDGE('',*,*,#14350,.T.);
#18971=ORIENTED_EDGE('',*,*,#14351,.T.);
#18972=ORIENTED_EDGE('',*,*,#14352,.T.);
#18973=ORIENTED_EDGE('',*,*,#14347,.T.);
#18974=ORIENTED_EDGE('',*,*,#14339,.T.);
#18975=ORIENTED_EDGE('',*,*,#14348,.F.);
#18976=ORIENTED_EDGE('',*,*,#14352,.F.);
#18977=ORIENTED_EDGE('',*,*,#14353,.T.);
#18978=ORIENTED_EDGE('',*,*,#14342,.F.);
#18979=ORIENTED_EDGE('',*,*,#14321,.F.);
#18980=ORIENTED_EDGE('',*,*,#14324,.F.);
#18981=ORIENTED_EDGE('',*,*,#14328,.F.);
#18982=ORIENTED_EDGE('',*,*,#14331,.F.);
#18983=ORIENTED_EDGE('',*,*,#14334,.F.);
#18984=ORIENTED_EDGE('',*,*,#14337,.F.);
#18985=ORIENTED_EDGE('',*,*,#14340,.F.);
#18986=ORIENTED_EDGE('',*,*,#14353,.F.);
#18987=ORIENTED_EDGE('',*,*,#14351,.F.);
#18988=ORIENTED_EDGE('',*,*,#14299,.F.);
#18989=ORIENTED_EDGE('',*,*,#14303,.F.);
#18990=ORIENTED_EDGE('',*,*,#14306,.F.);
#18991=ORIENTED_EDGE('',*,*,#14309,.F.);
#18992=ORIENTED_EDGE('',*,*,#14312,.F.);
#18993=ORIENTED_EDGE('',*,*,#14315,.F.);
#18994=ORIENTED_EDGE('',*,*,#14318,.F.);
#18995=ORIENTED_EDGE('',*,*,#14354,.F.);
#18996=ORIENTED_EDGE('',*,*,#14355,.F.);
#18997=ORIENTED_EDGE('',*,*,#14356,.F.);
#18998=ORIENTED_EDGE('',*,*,#14357,.F.);
#18999=ORIENTED_EDGE('',*,*,#14358,.F.);
#19000=ORIENTED_EDGE('',*,*,#14359,.F.);
#19001=ORIENTED_EDGE('',*,*,#14360,.F.);
#19002=ORIENTED_EDGE('',*,*,#14361,.F.);
#19003=ORIENTED_EDGE('',*,*,#14362,.F.);
#19004=ORIENTED_EDGE('',*,*,#14363,.F.);
#19005=ORIENTED_EDGE('',*,*,#14364,.F.);
#19006=ORIENTED_EDGE('',*,*,#14365,.F.);
#19007=ORIENTED_EDGE('',*,*,#14366,.F.);
#19008=ORIENTED_EDGE('',*,*,#14367,.T.);
#19009=ORIENTED_EDGE('',*,*,#14368,.F.);
#19010=ORIENTED_EDGE('',*,*,#14369,.F.);
#19011=ORIENTED_EDGE('',*,*,#14358,.T.);
#19012=ORIENTED_EDGE('',*,*,#14370,.F.);
#19013=ORIENTED_EDGE('',*,*,#14371,.F.);
#19014=ORIENTED_EDGE('',*,*,#14372,.F.);
#19015=ORIENTED_EDGE('',*,*,#14356,.T.);
#19016=ORIENTED_EDGE('',*,*,#14373,.F.);
#19017=ORIENTED_EDGE('',*,*,#14374,.F.);
#19018=ORIENTED_EDGE('',*,*,#14375,.F.);
#19019=ORIENTED_EDGE('',*,*,#14366,.T.);
#19020=ORIENTED_EDGE('',*,*,#14376,.F.);
#19021=ORIENTED_EDGE('',*,*,#14377,.F.);
#19022=ORIENTED_EDGE('',*,*,#14378,.F.);
#19023=ORIENTED_EDGE('',*,*,#14364,.T.);
#19024=ORIENTED_EDGE('',*,*,#14379,.F.);
#19025=ORIENTED_EDGE('',*,*,#14380,.F.);
#19026=ORIENTED_EDGE('',*,*,#14381,.F.);
#19027=ORIENTED_EDGE('',*,*,#14362,.T.);
#19028=ORIENTED_EDGE('',*,*,#14382,.F.);
#19029=ORIENTED_EDGE('',*,*,#14383,.F.);
#19030=ORIENTED_EDGE('',*,*,#14384,.F.);
#19031=ORIENTED_EDGE('',*,*,#14360,.T.);
#19032=ORIENTED_EDGE('',*,*,#14385,.F.);
#19033=ORIENTED_EDGE('',*,*,#14386,.F.);
#19034=ORIENTED_EDGE('',*,*,#14367,.F.);
#19035=ORIENTED_EDGE('',*,*,#14359,.T.);
#19036=ORIENTED_EDGE('',*,*,#14387,.F.);
#19037=ORIENTED_EDGE('',*,*,#14388,.F.);
#19038=ORIENTED_EDGE('',*,*,#14389,.T.);
#19039=ORIENTED_EDGE('',*,*,#14385,.T.);
#19040=ORIENTED_EDGE('',*,*,#14390,.T.);
#19041=ORIENTED_EDGE('',*,*,#14391,.T.);
#19042=ORIENTED_EDGE('',*,*,#14361,.T.);
#19043=ORIENTED_EDGE('',*,*,#14392,.F.);
#19044=ORIENTED_EDGE('',*,*,#14393,.F.);
#19045=ORIENTED_EDGE('',*,*,#14387,.T.);
#19046=ORIENTED_EDGE('',*,*,#14381,.T.);
#19047=ORIENTED_EDGE('',*,*,#14394,.T.);
#19048=ORIENTED_EDGE('',*,*,#14395,.F.);
#19049=ORIENTED_EDGE('',*,*,#14382,.T.);
#19050=ORIENTED_EDGE('',*,*,#14396,.T.);
#19051=ORIENTED_EDGE('',*,*,#14397,.T.);
#19052=ORIENTED_EDGE('',*,*,#14357,.T.);
#19053=ORIENTED_EDGE('',*,*,#14389,.F.);
#19054=ORIENTED_EDGE('',*,*,#14398,.F.);
#19055=ORIENTED_EDGE('',*,*,#14399,.T.);
#19056=ORIENTED_EDGE('',*,*,#14370,.T.);
#19057=ORIENTED_EDGE('',*,*,#14400,.T.);
#19058=ORIENTED_EDGE('',*,*,#14401,.T.);
#19059=ORIENTED_EDGE('',*,*,#14363,.T.);
#19060=ORIENTED_EDGE('',*,*,#14402,.F.);
#19061=ORIENTED_EDGE('',*,*,#14403,.F.);
#19062=ORIENTED_EDGE('',*,*,#14392,.T.);
#19063=ORIENTED_EDGE('',*,*,#14378,.T.);
#19064=ORIENTED_EDGE('',*,*,#14404,.T.);
#19065=ORIENTED_EDGE('',*,*,#14405,.F.);
#19066=ORIENTED_EDGE('',*,*,#14379,.T.);
#19067=ORIENTED_EDGE('',*,*,#14395,.T.);
#19068=ORIENTED_EDGE('',*,*,#14406,.T.);
#19069=ORIENTED_EDGE('',*,*,#14383,.T.);
#19070=ORIENTED_EDGE('',*,*,#14397,.F.);
#19071=ORIENTED_EDGE('',*,*,#14407,.F.);
#19072=ORIENTED_EDGE('',*,*,#14380,.T.);
#19073=ORIENTED_EDGE('',*,*,#14406,.F.);
#19074=ORIENTED_EDGE('',*,*,#14394,.F.);
#19075=ORIENTED_EDGE('',*,*,#14377,.T.);
#19076=ORIENTED_EDGE('',*,*,#14408,.F.);
#19077=ORIENTED_EDGE('',*,*,#14404,.F.);
#19078=ORIENTED_EDGE('',*,*,#14374,.T.);
#19079=ORIENTED_EDGE('',*,*,#14409,.F.);
#19080=ORIENTED_EDGE('',*,*,#14410,.F.);
#19081=ORIENTED_EDGE('',*,*,#14371,.T.);
#19082=ORIENTED_EDGE('',*,*,#14401,.F.);
#19083=ORIENTED_EDGE('',*,*,#14411,.F.);
#19084=ORIENTED_EDGE('',*,*,#14368,.T.);
#19085=ORIENTED_EDGE('',*,*,#14386,.T.);
#19086=ORIENTED_EDGE('',*,*,#14391,.F.);
#19087=ORIENTED_EDGE('',*,*,#14412,.F.);
#19088=ORIENTED_EDGE('',*,*,#14365,.T.);
#19089=ORIENTED_EDGE('',*,*,#14413,.F.);
#19090=ORIENTED_EDGE('',*,*,#14414,.F.);
#19091=ORIENTED_EDGE('',*,*,#14402,.T.);
#19092=ORIENTED_EDGE('',*,*,#14375,.T.);
#19093=ORIENTED_EDGE('',*,*,#14410,.T.);
#19094=ORIENTED_EDGE('',*,*,#14415,.F.);
#19095=ORIENTED_EDGE('',*,*,#14376,.T.);
#19096=ORIENTED_EDGE('',*,*,#14405,.T.);
#19097=ORIENTED_EDGE('',*,*,#14408,.T.);
#19098=ORIENTED_EDGE('',*,*,#14373,.T.);
#19099=ORIENTED_EDGE('',*,*,#14415,.T.);
#19100=ORIENTED_EDGE('',*,*,#14409,.T.);
#19101=ORIENTED_EDGE('',*,*,#14355,.T.);
#19102=ORIENTED_EDGE('',*,*,#14399,.F.);
#19103=ORIENTED_EDGE('',*,*,#14416,.F.);
#19104=ORIENTED_EDGE('',*,*,#14413,.T.);
#19105=ORIENTED_EDGE('',*,*,#14384,.T.);
#19106=ORIENTED_EDGE('',*,*,#14407,.T.);
#19107=ORIENTED_EDGE('',*,*,#14396,.F.);
#19108=ORIENTED_EDGE('',*,*,#14369,.T.);
#19109=ORIENTED_EDGE('',*,*,#14412,.T.);
#19110=ORIENTED_EDGE('',*,*,#14390,.F.);
#19111=ORIENTED_EDGE('',*,*,#14372,.T.);
#19112=ORIENTED_EDGE('',*,*,#14411,.T.);
#19113=ORIENTED_EDGE('',*,*,#14400,.F.);
#19114=ORIENTED_EDGE('',*,*,#14417,.F.);
#19115=ORIENTED_EDGE('',*,*,#14349,.F.);
#19116=ORIENTED_EDGE('',*,*,#14300,.F.);
#19117=ORIENTED_EDGE('',*,*,#14350,.F.);
#19118=ORIENTED_EDGE('',*,*,#14418,.T.);
#19119=ORIENTED_EDGE('',*,*,#14417,.T.);
#19120=ORIENTED_EDGE('',*,*,#14418,.F.);
#19121=ORIENTED_EDGE('',*,*,#14317,.T.);
#19122=ORIENTED_EDGE('',*,*,#14346,.T.);
#19123=ORIENTED_EDGE('',*,*,#14419,.F.);
#19124=ORIENTED_EDGE('',*,*,#14354,.T.);
#19125=ORIENTED_EDGE('',*,*,#14420,.F.);
#19126=ORIENTED_EDGE('',*,*,#14421,.T.);
#19127=ORIENTED_EDGE('',*,*,#14343,.T.);
#19128=ORIENTED_EDGE('',*,*,#14419,.T.);
#19129=ORIENTED_EDGE('',*,*,#14344,.T.);
#19130=ORIENTED_EDGE('',*,*,#14421,.F.);
#19131=ORIENTED_EDGE('',*,*,#14420,.T.);
#19132=ORIENTED_EDGE('',*,*,#14403,.T.);
#19133=ORIENTED_EDGE('',*,*,#14414,.T.);
#19134=ORIENTED_EDGE('',*,*,#14416,.T.);
#19135=ORIENTED_EDGE('',*,*,#14398,.T.);
#19136=ORIENTED_EDGE('',*,*,#14388,.T.);
#19137=ORIENTED_EDGE('',*,*,#14393,.T.);
#25327=CONICAL_SURFACE('',#27470,0.288675134594813,1.02910423288134);
#25328=CONICAL_SURFACE('',#27504,0.875,0.785398163397448);
#25329=CONICAL_SURFACE('',#27507,0.96,0.785398163397449);
#25634=ADVANCED_FACE('',(#2821),#606,.T.);
#25635=ADVANCED_FACE('',(#2822),#607,.T.);
#25636=ADVANCED_FACE('',(#2823),#608,.T.);
#25637=ADVANCED_FACE('',(#2824),#609,.T.);
#25638=ADVANCED_FACE('',(#2825),#610,.T.);
#25639=ADVANCED_FACE('',(#2826),#611,.T.);
#25640=ADVANCED_FACE('',(#2827),#612,.T.);
#25641=ADVANCED_FACE('',(#2828),#613,.T.);
#25642=ADVANCED_FACE('',(#2829),#614,.T.);
#25643=ADVANCED_FACE('',(#2830),#615,.T.);
#25644=ADVANCED_FACE('',(#2831),#616,.T.);
#25645=ADVANCED_FACE('',(#2832),#617,.T.);
#25646=ADVANCED_FACE('',(#2833),#618,.T.);
#25647=ADVANCED_FACE('',(#2834),#619,.T.);
#25648=ADVANCED_FACE('',(#2835),#1765,.F.);
#25649=ADVANCED_FACE('',(#2836),#274,.F.);
#25650=ADVANCED_FACE('',(#2837),#1766,.T.);
#25651=ADVANCED_FACE('',(#2838),#620,.T.);
#25652=ADVANCED_FACE('',(#2839),#275,.F.);
#25653=ADVANCED_FACE('',(#2840),#1767,.F.);
#25654=ADVANCED_FACE('',(#2841),#1768,.F.);
#25655=ADVANCED_FACE('',(#2842),#1769,.F.);
#25656=ADVANCED_FACE('',(#2843),#1770,.F.);
#25657=ADVANCED_FACE('',(#2844),#1771,.F.);
#25658=ADVANCED_FACE('',(#2845),#1772,.F.);
#25659=ADVANCED_FACE('',(#2846),#25327,.F.);
#25660=ADVANCED_FACE('',(#2847),#1773,.F.);
#25661=ADVANCED_FACE('',(#2848),#1774,.F.);
#25662=ADVANCED_FACE('',(#2849),#1775,.F.);
#25663=ADVANCED_FACE('',(#2850),#1776,.F.);
#25664=ADVANCED_FACE('',(#2851),#1777,.F.);
#25665=ADVANCED_FACE('',(#2852),#1778,.F.);
#25666=ADVANCED_FACE('',(#2853),#1779,.F.);
#25667=ADVANCED_FACE('',(#2854),#1780,.F.);
#25668=ADVANCED_FACE('',(#2855),#1781,.F.);
#25669=ADVANCED_FACE('',(#2856),#1782,.F.);
#25670=ADVANCED_FACE('',(#2857),#1783,.F.);
#25671=ADVANCED_FACE('',(#2858),#1784,.F.);
#25672=ADVANCED_FACE('',(#2859),#1785,.F.);
#25673=ADVANCED_FACE('',(#2860),#1786,.F.);
#25674=ADVANCED_FACE('',(#2861),#1787,.F.);
#25675=ADVANCED_FACE('',(#2862),#1788,.F.);
#25676=ADVANCED_FACE('',(#2863),#1789,.F.);
#25677=ADVANCED_FACE('',(#2864),#1790,.F.);
#25678=ADVANCED_FACE('',(#2865),#1791,.F.);
#25679=ADVANCED_FACE('',(#2866),#1792,.F.);
#25680=ADVANCED_FACE('',(#2867),#1793,.F.);
#25681=ADVANCED_FACE('',(#2868),#1794,.F.);
#25682=ADVANCED_FACE('',(#2869),#1795,.F.);
#25683=ADVANCED_FACE('',(#2870),#1796,.F.);
#25684=ADVANCED_FACE('',(#2871),#1797,.T.);
#25685=ADVANCED_FACE('',(#2872),#25328,.T.);
#25686=ADVANCED_FACE('',(#2873),#621,.T.);
#25687=ADVANCED_FACE('',(#2874),#25329,.T.);
#25688=ADVANCED_FACE('',(#2875,#861),#1798,.T.);
#26877=CLOSED_SHELL('',(#25634,#25635,#25636,#25637,#25638,#25639,#25640,
#25641,#25642,#25643,#25644,#25645,#25646,#25647,#25648,#25649,#25650,#25651,
#25652,#25653,#25654,#25655,#25656,#25657,#25658,#25659,#25660,#25661,#25662,
#25663,#25664,#25665,#25666,#25667,#25668,#25669,#25670,#25671,#25672,#25673,
#25674,#25675,#25676,#25677,#25678,#25679,#25680,#25681,#25682,#25683,#25684,
#25685,#25686,#25687,#25688));
#27432=AXIS2_PLACEMENT_3D('',#45342,#30037,#30038);
#27433=AXIS2_PLACEMENT_3D('',#45343,#30039,#30040);
#27434=AXIS2_PLACEMENT_3D('',#45365,#30042,#30043);
#27435=AXIS2_PLACEMENT_3D('',#45376,#30044,#30045);
#27436=AXIS2_PLACEMENT_3D('',#45460,#30047,#30048);
#27437=AXIS2_PLACEMENT_3D('',#45550,#30050,#30051);
#27438=AXIS2_PLACEMENT_3D('',#45640,#30053,#30054);
#27439=AXIS2_PLACEMENT_3D('',#45730,#30056,#30057);
#27440=AXIS2_PLACEMENT_3D('',#45814,#30059,#30060);
#27441=AXIS2_PLACEMENT_3D('',#45904,#30062,#30063);
#27442=AXIS2_PLACEMENT_3D('',#45914,#30065,#30066);
#27443=AXIS2_PLACEMENT_3D('',#45915,#30067,#30068);
#27444=AXIS2_PLACEMENT_3D('',#45937,#30070,#30071);
#27445=AXIS2_PLACEMENT_3D('',#45953,#30072,#30073);
#27446=AXIS2_PLACEMENT_3D('',#45990,#30075,#30076);
#27447=AXIS2_PLACEMENT_3D('',#46027,#30078,#30079);
#27448=AXIS2_PLACEMENT_3D('',#46065,#30081,#30082);
#27449=AXIS2_PLACEMENT_3D('',#46103,#30084,#30085);
#27450=AXIS2_PLACEMENT_3D('',#46140,#30087,#30088);
#27451=AXIS2_PLACEMENT_3D('',#46219,#30089,#30090);
#27452=AXIS2_PLACEMENT_3D('',#46221,#30091,#30092);
#27453=AXIS2_PLACEMENT_3D('',#46789,#30093,#30094);
#27454=AXIS2_PLACEMENT_3D('',#46791,#30095,#30096);
#27455=AXIS2_PLACEMENT_3D('',#46792,#30097,#30098);
#27456=AXIS2_PLACEMENT_3D('',#46873,#30099,#30100);
#27457=AXIS2_PLACEMENT_3D('',#46874,#30101,#30102);
#27458=AXIS2_PLACEMENT_3D('',#47278,#30103,#30104);
#27459=AXIS2_PLACEMENT_3D('',#47282,#30106,#30107);
#27460=AXIS2_PLACEMENT_3D('',#47283,#30108,#30109);
#27461=AXIS2_PLACEMENT_3D('',#47286,#30111,#30112);
#27462=AXIS2_PLACEMENT_3D('',#47287,#30113,#30114);
#27463=AXIS2_PLACEMENT_3D('',#47290,#30116,#30117);
#27464=AXIS2_PLACEMENT_3D('',#47291,#30118,#30119);
#27465=AXIS2_PLACEMENT_3D('',#47294,#30121,#30122);
#27466=AXIS2_PLACEMENT_3D('',#47295,#30123,#30124);
#27467=AXIS2_PLACEMENT_3D('',#47298,#30126,#30127);
#27468=AXIS2_PLACEMENT_3D('',#47299,#30128,#30129);
#27469=AXIS2_PLACEMENT_3D('',#47301,#30131,#30132);
#27470=AXIS2_PLACEMENT_3D('',#47302,#30133,#30134);
#27471=AXIS2_PLACEMENT_3D('',#47307,#30136,#30137);
#27472=AXIS2_PLACEMENT_3D('',#47316,#30138,#30139);
#27473=AXIS2_PLACEMENT_3D('',#47325,#30140,#30141);
#27474=AXIS2_PLACEMENT_3D('',#47334,#30142,#30143);
#27475=AXIS2_PLACEMENT_3D('',#47343,#30144,#30145);
#27476=AXIS2_PLACEMENT_3D('',#47352,#30146,#30147);
#27477=AXIS2_PLACEMENT_3D('',#47360,#30148,#30149);
#27478=AXIS2_PLACEMENT_3D('',#47361,#30150,#30151);
#27479=AXIS2_PLACEMENT_3D('',#47367,#30155,#30156);
#27480=AXIS2_PLACEMENT_3D('',#47371,#30159,#30160);
#27481=AXIS2_PLACEMENT_3D('',#47375,#30163,#30164);
#27482=AXIS2_PLACEMENT_3D('',#47379,#30167,#30168);
#27483=AXIS2_PLACEMENT_3D('',#47383,#30171,#30172);
#27484=AXIS2_PLACEMENT_3D('',#47387,#30175,#30176);
#27485=AXIS2_PLACEMENT_3D('',#47391,#30179,#30180);
#27486=AXIS2_PLACEMENT_3D('',#47395,#30183,#30184);
#27487=AXIS2_PLACEMENT_3D('',#47399,#30187,#30188);
#27488=AXIS2_PLACEMENT_3D('',#47401,#30190,#30191);
#27489=AXIS2_PLACEMENT_3D('',#47403,#30193,#30194);
#27490=AXIS2_PLACEMENT_3D('',#47404,#30195,#30196);
#27491=AXIS2_PLACEMENT_3D('',#47406,#30198,#30199);
#27492=AXIS2_PLACEMENT_3D('',#47410,#30202,#30203);
#27493=AXIS2_PLACEMENT_3D('',#47412,#30205,#30206);
#27494=AXIS2_PLACEMENT_3D('',#47414,#30208,#30209);
#27495=AXIS2_PLACEMENT_3D('',#47418,#30212,#30213);
#27496=AXIS2_PLACEMENT_3D('',#47420,#30215,#30216);
#27497=AXIS2_PLACEMENT_3D('',#47421,#30217,#30218);
#27498=AXIS2_PLACEMENT_3D('',#47422,#30219,#30220);
#27499=AXIS2_PLACEMENT_3D('',#47424,#30222,#30223);
#27500=AXIS2_PLACEMENT_3D('',#47425,#30224,#30225);
#27501=AXIS2_PLACEMENT_3D('',#47426,#30226,#30227);
#27502=AXIS2_PLACEMENT_3D('',#47427,#30228,#30229);
#27503=AXIS2_PLACEMENT_3D('',#47429,#30230,#30231);
#27504=AXIS2_PLACEMENT_3D('',#47430,#30232,#30233);
#27505=AXIS2_PLACEMENT_3D('',#47432,#30235,#30236);
#27506=AXIS2_PLACEMENT_3D('',#47433,#30237,#30238);
#27507=AXIS2_PLACEMENT_3D('',#47434,#30239,#30240);
#27508=AXIS2_PLACEMENT_3D('',#47436,#30241,#30242);
#27509=AXIS2_PLACEMENT_3D('',#47438,#30244,#30245);
#30037=DIRECTION('axis',(0.,0.,1.));
#30038=DIRECTION('refdir',(1.,0.,0.));
#30039=DIRECTION('center_axis',(0.,0.,1.));
#30040=DIRECTION('ref_axis',(1.,0.,0.));
#30041=DIRECTION('',(0.,0.,-1.));
#30042=DIRECTION('center_axis',(0.,0.,1.));
#30043=DIRECTION('ref_axis',(1.,0.,0.));
#30044=DIRECTION('center_axis',(0.,0.,1.));
#30045=DIRECTION('ref_axis',(1.,0.,0.));
#30046=DIRECTION('',(0.,0.,-1.));
#30047=DIRECTION('center_axis',(0.,0.,1.));
#30048=DIRECTION('ref_axis',(1.,0.,0.));
#30049=DIRECTION('',(0.,0.,-1.));
#30050=DIRECTION('center_axis',(0.,0.,1.));
#30051=DIRECTION('ref_axis',(1.,0.,0.));
#30052=DIRECTION('',(0.,0.,-1.));
#30053=DIRECTION('center_axis',(0.,0.,1.));
#30054=DIRECTION('ref_axis',(1.,0.,0.));
#30055=DIRECTION('',(0.,0.,-1.));
#30056=DIRECTION('center_axis',(0.,0.,1.));
#30057=DIRECTION('ref_axis',(1.,0.,0.));
#30058=DIRECTION('',(0.,0.,-1.));
#30059=DIRECTION('center_axis',(0.,0.,1.));
#30060=DIRECTION('ref_axis',(1.,0.,0.));
#30061=DIRECTION('',(0.,0.,-1.));
#30062=DIRECTION('center_axis',(0.,0.,1.));
#30063=DIRECTION('ref_axis',(-0.938278381435466,-0.345881018459878,0.));
#30064=DIRECTION('',(0.,0.,1.));
#30065=DIRECTION('center_axis',(0.,0.,1.));
#30066=DIRECTION('ref_axis',(1.,2.10412784742716E-14,0.));
#30067=DIRECTION('center_axis',(0.,0.,1.));
#30068=DIRECTION('ref_axis',(1.,2.10412784742716E-14,0.));
#30069=DIRECTION('',(0.,0.,1.));
#30070=DIRECTION('center_axis',(0.,0.,1.));
#30071=DIRECTION('ref_axis',(1.,2.10412784742716E-14,0.));
#30072=DIRECTION('center_axis',(0.,0.,1.));
#30073=DIRECTION('ref_axis',(1.,2.10412784742716E-14,0.));
#30074=DIRECTION('',(0.,0.,1.));
#30075=DIRECTION('center_axis',(0.,0.,1.));
#30076=DIRECTION('ref_axis',(1.,2.10412784742716E-14,0.));
#30077=DIRECTION('',(0.,0.,1.));
#30078=DIRECTION('center_axis',(0.,0.,1.));
#30079=DIRECTION('ref_axis',(1.,2.10412784742716E-14,0.));
#30080=DIRECTION('',(0.,0.,1.));
#30081=DIRECTION('center_axis',(0.,0.,1.));
#30082=DIRECTION('ref_axis',(1.,2.10412784742716E-14,0.));
#30083=DIRECTION('',(0.,0.,1.));
#30084=DIRECTION('center_axis',(0.,0.,1.));
#30085=DIRECTION('ref_axis',(1.,2.10412784742716E-14,0.));
#30086=DIRECTION('',(0.,0.,1.));
#30087=DIRECTION('center_axis',(0.,0.,1.));
#30088=DIRECTION('ref_axis',(1.,0.,0.));
#30089=DIRECTION('center_axis',(0.,0.,-1.));
#30090=DIRECTION('ref_axis',(1.,0.,0.));
#30091=DIRECTION('center_axis',(0.,0.,-1.));
#30092=DIRECTION('ref_axis',(1.,0.,0.));
#30093=DIRECTION('center_axis',(0.,0.,1.));
#30094=DIRECTION('ref_axis',(1.,0.,0.));
#30095=DIRECTION('center_axis',(0.,0.,1.));
#30096=DIRECTION('ref_axis',(1.,0.,0.));
#30097=DIRECTION('center_axis',(0.,0.,1.));
#30098=DIRECTION('ref_axis',(1.,0.,0.));
#30099=DIRECTION('center_axis',(0.,0.,-1.));
#30100=DIRECTION('ref_axis',(1.,2.10412784742716E-14,0.));
#30101=DIRECTION('center_axis',(0.,0.,1.));
#30102=DIRECTION('ref_axis',(0.88903119899841,0.457846619740114,0.));
#30103=DIRECTION('center_axis',(0.,0.,1.));
#30104=DIRECTION('ref_axis',(1.,0.,0.));
#30105=DIRECTION('',(-1.,1.92296268638356E-16,0.));
#30106=DIRECTION('center_axis',(0.,0.,1.));
#30107=DIRECTION('ref_axis',(1.,0.,0.));
#30108=DIRECTION('center_axis',(0.,0.,1.));
#30109=DIRECTION('ref_axis',(1.,0.,0.));
#30110=DIRECTION('',(-0.5,0.866025403784439,0.));
#30111=DIRECTION('center_axis',(0.,0.,1.));
#30112=DIRECTION('ref_axis',(1.,0.,0.));
#30113=DIRECTION('center_axis',(0.,0.,1.));
#30114=DIRECTION('ref_axis',(1.,0.,0.));
#30115=DIRECTION('',(0.5,0.866025403784438,0.));
#30116=DIRECTION('center_axis',(0.,0.,1.));
#30117=DIRECTION('ref_axis',(1.,0.,0.));
#30118=DIRECTION('center_axis',(0.,0.,1.));
#30119=DIRECTION('ref_axis',(1.,0.,0.));
#30120=DIRECTION('',(1.,-1.92296268638356E-16,0.));
#30121=DIRECTION('center_axis',(0.,0.,1.));
#30122=DIRECTION('ref_axis',(1.,0.,0.));
#30123=DIRECTION('center_axis',(0.,0.,1.));
#30124=DIRECTION('ref_axis',(1.,0.,0.));
#30125=DIRECTION('',(0.5,-0.866025403784439,0.));
#30126=DIRECTION('center_axis',(0.,0.,1.));
#30127=DIRECTION('ref_axis',(1.,0.,0.));
#30128=DIRECTION('center_axis',(0.,0.,1.));
#30129=DIRECTION('ref_axis',(1.,0.,0.));
#30130=DIRECTION('',(-0.5,-0.866025403784439,0.));
#30131=DIRECTION('center_axis',(0.,0.,1.));
#30132=DIRECTION('ref_axis',(1.,0.,0.));
#30133=DIRECTION('center_axis',(0.,0.,1.));
#30134=DIRECTION('ref_axis',(1.,0.,0.));
#30135=DIRECTION('',(-0.856837487509096,-1.04932328646748E-16,0.515586578567653));
#30136=DIRECTION('center_axis',(0.,0.,-1.));
#30137=DIRECTION('ref_axis',(1.,0.,0.));
#30138=DIRECTION('center_axis',(0.,0.,-1.));
#30139=DIRECTION('ref_axis',(1.,0.,0.));
#30140=DIRECTION('center_axis',(0.,0.,-1.));
#30141=DIRECTION('ref_axis',(1.,0.,0.));
#30142=DIRECTION('center_axis',(0.,0.,-1.));
#30143=DIRECTION('ref_axis',(1.,0.,0.));
#30144=DIRECTION('center_axis',(0.,0.,-1.));
#30145=DIRECTION('ref_axis',(1.,0.,0.));
#30146=DIRECTION('center_axis',(0.,0.,-1.));
#30147=DIRECTION('ref_axis',(1.,0.,0.));
#30148=DIRECTION('center_axis',(0.,0.,-1.));
#30149=DIRECTION('ref_axis',(1.,0.,0.));
#30150=DIRECTION('center_axis',(-0.866025403784438,0.5,0.));
#30151=DIRECTION('ref_axis',(0.5,0.866025403784438,0.));
#30152=DIRECTION('',(0.,0.,-1.));
#30153=DIRECTION('',(0.5,0.866025403784438,0.));
#30154=DIRECTION('',(0.,0.,-1.));
#30155=DIRECTION('center_axis',(-0.866025403784438,0.5,0.));
#30156=DIRECTION('ref_axis',(0.5,0.866025403784438,0.));
#30157=DIRECTION('',(0.,0.,-1.));
#30158=DIRECTION('',(0.5,0.866025403784438,0.));
#30159=DIRECTION('center_axis',(1.92296268638356E-16,1.,0.));
#30160=DIRECTION('ref_axis',(1.,-1.92296268638356E-16,0.));
#30161=DIRECTION('',(0.,0.,-1.));
#30162=DIRECTION('',(1.,-1.92296268638356E-16,0.));
#30163=DIRECTION('center_axis',(1.92296268638356E-16,1.,0.));
#30164=DIRECTION('ref_axis',(1.,-1.92296268638356E-16,0.));
#30165=DIRECTION('',(1.,-1.92296268638356E-16,0.));
#30166=DIRECTION('',(0.,0.,-1.));
#30167=DIRECTION('center_axis',(1.92296268638356E-16,1.,0.));
#30168=DIRECTION('ref_axis',(1.,-1.92296268638356E-16,0.));
#30169=DIRECTION('',(0.,0.,-1.));
#30170=DIRECTION('',(1.,-1.92296268638356E-16,0.));
#30171=DIRECTION('center_axis',(-0.866025403784439,-0.5,0.));
#30172=DIRECTION('ref_axis',(-0.5,0.866025403784439,0.));
#30173=DIRECTION('',(-0.5,0.866025403784439,0.));
#30174=DIRECTION('',(0.,0.,-1.));
#30175=DIRECTION('center_axis',(-0.866025403784439,-0.5,0.));
#30176=DIRECTION('ref_axis',(-0.5,0.866025403784439,0.));
#30177=DIRECTION('',(0.,0.,-1.));
#30178=DIRECTION('',(-0.5,0.866025403784439,0.));
#30179=DIRECTION('center_axis',(0.866025403784439,0.5,0.));
#30180=DIRECTION('ref_axis',(0.5,-0.866025403784439,0.));
#30181=DIRECTION('',(0.,0.,-1.));
#30182=DIRECTION('',(0.5,-0.866025403784439,0.));
#30183=DIRECTION('center_axis',(0.866025403784439,0.5,0.));
#30184=DIRECTION('ref_axis',(0.5,-0.866025403784439,0.));
#30185=DIRECTION('',(0.5,-0.866025403784439,0.));
#30186=DIRECTION('',(0.,0.,-1.));
#30187=DIRECTION('center_axis',(0.866025403784439,0.5,0.));
#30188=DIRECTION('ref_axis',(0.5,-0.866025403784439,0.));
#30189=DIRECTION('',(0.5,-0.866025403784439,0.));
#30190=DIRECTION('center_axis',(0.,0.,-1.));
#30191=DIRECTION('ref_axis',(-1.,0.,0.));
#30192=DIRECTION('',(0.5,0.866025403784438,0.));
#30193=DIRECTION('center_axis',(0.,0.,-1.));
#30194=DIRECTION('ref_axis',(-1.,0.,0.));
#30195=DIRECTION('center_axis',(0.,0.,-1.));
#30196=DIRECTION('ref_axis',(-1.,0.,0.));
#30197=DIRECTION('',(-0.5,-0.866025403784439,0.));
#30198=DIRECTION('center_axis',(0.,0.,-1.));
#30199=DIRECTION('ref_axis',(-1.,0.,0.));
#30200=DIRECTION('',(-1.,1.92296268638356E-16,0.));
#30201=DIRECTION('',(-0.5,-0.866025403784439,0.));
#30202=DIRECTION('center_axis',(0.,0.,-1.));
#30203=DIRECTION('ref_axis',(-1.,0.,0.));
#30204=DIRECTION('',(-1.,1.92296268638356E-16,0.));
#30205=DIRECTION('center_axis',(0.,0.,-1.));
#30206=DIRECTION('ref_axis',(-1.,0.,0.));
#30207=DIRECTION('',(-0.5,0.866025403784439,0.));
#30208=DIRECTION('center_axis',(0.866025403784439,-0.5,0.));
#30209=DIRECTION('ref_axis',(-0.5,-0.866025403784439,0.));
#30210=DIRECTION('',(0.,0.,-1.));
#30211=DIRECTION('',(-0.5,-0.866025403784439,0.));
#30212=DIRECTION('center_axis',(0.866025403784439,-0.5,0.));
#30213=DIRECTION('ref_axis',(-0.5,-0.866025403784439,0.));
#30214=DIRECTION('',(0.,0.,-1.));
#30215=DIRECTION('center_axis',(0.866025403784439,-0.5,0.));
#30216=DIRECTION('ref_axis',(-0.5,-0.866025403784439,0.));
#30217=DIRECTION('center_axis',(-1.92296268638356E-16,-1.,0.));
#30218=DIRECTION('ref_axis',(-1.,1.92296268638356E-16,0.));
#30219=DIRECTION('center_axis',(-1.92296268638356E-16,-1.,0.));
#30220=DIRECTION('ref_axis',(-1.,1.92296268638356E-16,0.));
#30221=DIRECTION('',(-1.,1.92296268638356E-16,0.));
#30222=DIRECTION('center_axis',(-0.866025403784438,0.5,0.));
#30223=DIRECTION('ref_axis',(0.5,0.866025403784438,0.));
#30224=DIRECTION('center_axis',(-0.866025403784439,-0.5,0.));
#30225=DIRECTION('ref_axis',(-0.5,0.866025403784439,0.));
#30226=DIRECTION('center_axis',(-1.92296268638356E-16,-1.,0.));
#30227=DIRECTION('ref_axis',(-1.,1.92296268638356E-16,0.));
#30228=DIRECTION('center_axis',(0.,0.,-1.));
#30229=DIRECTION('ref_axis',(-1.,0.,0.));
#30230=DIRECTION('center_axis',(0.,0.,1.));
#30231=DIRECTION('ref_axis',(1.,0.,0.));
#30232=DIRECTION('center_axis',(0.,0.,1.));
#30233=DIRECTION('ref_axis',(1.,0.,0.));
#30234=DIRECTION('',(0.707106781186548,8.65956056235493E-17,-0.707106781186547));
#30235=DIRECTION('center_axis',(0.,0.,1.));
#30236=DIRECTION('ref_axis',(0.266308421152316,-0.963887869424323,0.));
#30237=DIRECTION('center_axis',(0.,0.,-1.));
#30238=DIRECTION('ref_axis',(1.,0.,0.));
#30239=DIRECTION('center_axis',(0.,0.,-1.));
#30240=DIRECTION('ref_axis',(1.,0.,0.));
#30241=DIRECTION('center_axis',(0.,0.,1.));
#30242=DIRECTION('ref_axis',(1.,0.,0.));
#30243=DIRECTION('',(-0.707106781186548,-8.65956056235494E-17,-0.707106781186547));
#30244=DIRECTION('center_axis',(0.,0.,1.));
#30245=DIRECTION('ref_axis',(1.,0.,0.));
#45342=CARTESIAN_POINT('',(0.,0.,0.));
#45343=CARTESIAN_POINT('Origin',(0.,0.,-0.915));
#45344=CARTESIAN_POINT('',(-0.989508121607439,2.46417016753209E-5,-1.67997427199779));
#45345=CARTESIAN_POINT('',(-0.989512555708751,1.62595781710845E-5,-1.71597572800221));
#45346=CARTESIAN_POINT('',(-0.989525,-1.21181862392628E-16,-0.915));
#45347=CARTESIAN_POINT('',(0.432569264169048,0.889983862027826,-1.760475));
#45348=CARTESIAN_POINT('Ctrl Pts',(-0.989508121607439,2.46417016753209E-5,
-1.67997427199779));
#45349=CARTESIAN_POINT('Ctrl Pts',(-0.989549791832843,0.0432915798739707,
-1.68171398035312));
#45350=CARTESIAN_POINT('Ctrl Pts',(-0.986763738908389,0.0865531766282412,
-1.68345368870845));
#45351=CARTESIAN_POINT('Ctrl Pts',(-0.981106280255709,0.129435929606698,
-1.68519339706378));
#45352=CARTESIAN_POINT('Ctrl Pts',(-0.959748207461145,0.291327163104516,
-1.69176115477542));
#45353=CARTESIAN_POINT('Ctrl Pts',(-0.897466338773216,0.447819046310428,
-1.69832891248706));
#45354=CARTESIAN_POINT('Ctrl Pts',(-0.801742294532236,0.580113943815296,
-1.7048966701987));
#45355=CARTESIAN_POINT('Ctrl Pts',(-0.706018250291256,0.712408841320163,
-1.71146442791034));
#45356=CARTESIAN_POINT('Ctrl Pts',(-0.576852030497224,0.820506753123986,
-1.71803218562198));
#45357=CARTESIAN_POINT('Ctrl Pts',(-0.429759709431166,0.891420527045617,
-1.72459994333363));
#45358=CARTESIAN_POINT('Ctrl Pts',(-0.282667388365107,0.962334300967249,
-1.73116770104527));
#45359=CARTESIAN_POINT('Ctrl Pts',(-0.117648966027021,0.99606393700669,
-1.73773545875691));
#45360=CARTESIAN_POINT('Ctrl Pts',(0.0454726780246543,0.988561401513198,
-1.74430321646855));
#45361=CARTESIAN_POINT('Ctrl Pts',(0.179357434066637,0.982403572856662,
-1.74969381097903));
#45362=CARTESIAN_POINT('Ctrl Pts',(0.311964411384094,0.948469386821795,
-1.75508440548952));
#45363=CARTESIAN_POINT('Ctrl Pts',(0.4325852656532,0.88999165664392,-1.760475));
#45364=CARTESIAN_POINT('',(-0.4325532626849,0.88997606741173,-1.760475));
#45365=CARTESIAN_POINT('Origin',(0.,0.,-1.760475));
#45366=CARTESIAN_POINT('Ctrl Pts',(-0.4325532626849,0.88997606741173,-1.760475));
#45367=CARTESIAN_POINT('Ctrl Pts',(-0.579457834201592,0.818576336520455,
-1.75390724228836));
#45368=CARTESIAN_POINT('Ctrl Pts',(-0.708275027509353,0.710144989051779,
-1.74733948457672));
#45369=CARTESIAN_POINT('Ctrl Pts',(-0.803577819756788,0.577570371582787,
-1.74077172686507));
#45370=CARTESIAN_POINT('Ctrl Pts',(-0.898880612004223,0.444995754113794,
-1.73420396915343));
#45371=CARTESIAN_POINT('Ctrl Pts',(-0.960669003191333,0.288277866644485,
-1.72763621144179));
#45372=CARTESIAN_POINT('Ctrl Pts',(-0.981513623068095,0.126312099804374,
-1.72106845373015));
#45373=CARTESIAN_POINT('Ctrl Pts',(-0.986901353888686,0.0844486377194643,
-1.7193708784875));
#45374=CARTESIAN_POINT('Ctrl Pts',(-0.989553742529366,0.0422345790642187,
-1.71767330324486));
#45375=CARTESIAN_POINT('Ctrl Pts',(-0.989512555708751,1.62595781710845E-5,
-1.71597572800221));
#45376=CARTESIAN_POINT('Origin',(0.,0.,-0.915));
#45377=CARTESIAN_POINT('',(-0.989602407284016,-7.73947795529306E-6,-1.42997427199779));
#45378=CARTESIAN_POINT('',(-0.989600974548901,-8.74702472718336E-6,-1.46597572800221));
#45379=CARTESIAN_POINT('',(-0.989525,-1.21181862392628E-16,-0.915));
#45380=CARTESIAN_POINT('Ctrl Pts',(-0.989602407284016,-7.73947795529306E-6,
-1.42997427199779));
#45381=CARTESIAN_POINT('Ctrl Pts',(-0.989536830744615,0.155635723124492,
-1.43623422114676));
#45382=CARTESIAN_POINT('Ctrl Pts',(-0.952173126552117,0.311309569170158,
-1.44249417029572));
#45383=CARTESIAN_POINT('Ctrl Pts',(-0.881409540624574,0.449933753797064,
-1.44875411944469));
#45384=CARTESIAN_POINT('Ctrl Pts',(-0.807166431596158,0.595374241561052,
-1.45532187715633));
#45385=CARTESIAN_POINT('Ctrl Pts',(-0.696158069103402,0.722047144202599,
-1.46188963486797));
#45386=CARTESIAN_POINT('Ctrl Pts',(-0.561719334295483,0.814735877727747,
-1.46845739257961));
#45387=CARTESIAN_POINT('Ctrl Pts',(-0.427280599487563,0.907424611252896,
-1.47502515029125));
#45388=CARTESIAN_POINT('Ctrl Pts',(-0.26941149236448,0.966129175661646,
-1.48159290800289));
#45389=CARTESIAN_POINT('Ctrl Pts',(-0.107076041692171,0.983797683784885,
-1.48816066571454));
#45390=CARTESIAN_POINT('Ctrl Pts',(0.0552594089801381,1.00146619190812,
-1.49472842342618));
#45391=CARTESIAN_POINT('Ctrl Pts',(0.222061203201673,0.978098643745851,
-1.50129618113782));
#45392=CARTESIAN_POINT('Ctrl Pts',(0.373292273023635,0.916502067392168,
-1.50786393884946));
#45393=CARTESIAN_POINT('Ctrl Pts',(0.524523342845598,0.854905491038486,
-1.5144316965611));
#45394=CARTESIAN_POINT('Ctrl Pts',(0.660183688267988,0.755079886493395,
-1.52099945427274));
#45395=CARTESIAN_POINT('Ctrl Pts',(0.763977108360576,0.629016803897046,
-1.52756721198439));
#45396=CARTESIAN_POINT('Ctrl Pts',(0.867770528453163,0.502953721300697,
-1.53413496969603));
#45397=CARTESIAN_POINT('Ctrl Pts',(0.939697023215948,0.350653160653091,
-1.54070272740767));
#45398=CARTESIAN_POINT('Ctrl Pts',(0.971116421385275,0.190410233050476,
-1.54727048511931));
#45399=CARTESIAN_POINT('Ctrl Pts',(1.0025358195546,0.0301673054478622,-1.55383824283095));
#45400=CARTESIAN_POINT('Ctrl Pts',(0.99344812113047,-0.13801798910976,-1.56040600054259));
#45401=CARTESIAN_POINT('Ctrl Pts',(0.944944986100939,-0.29394239770406,
-1.56697375825423));
#45402=CARTESIAN_POINT('Ctrl Pts',(0.896441851071408,-0.44986680629836,
-1.57354151596587));
#45403=CARTESIAN_POINT('Ctrl Pts',(0.808523279436478,-0.593530328929339,
-1.58010927367752));
#45404=CARTESIAN_POINT('Ctrl Pts',(0.691750490716862,-0.707675366998289,
-1.58667703138916));
#45405=CARTESIAN_POINT('Ctrl Pts',(0.574977701997246,-0.821820405067239,
-1.5932447891008));
#45406=CARTESIAN_POINT('Ctrl Pts',(0.429350696192944,-0.906446958574161,
-1.59981254681244));
#45407=CARTESIAN_POINT('Ctrl Pts',(0.272362919805735,-0.951389292968879,
-1.60638030452408));
#45408=CARTESIAN_POINT('Ctrl Pts',(0.115375143418526,-0.996331627363596,
-1.61294806223572));
#45409=CARTESIAN_POINT('Ctrl Pts',(-0.0529734035515899,-1.00158974264611,
-1.61951581994736));
#45410=CARTESIAN_POINT('Ctrl Pts',(-0.212459850119537,-0.966531945468779,
-1.62608357765901));
#45411=CARTESIAN_POINT('Ctrl Pts',(-0.371946296687484,-0.93147414829145,
-1.63265133537065));
#45412=CARTESIAN_POINT('Ctrl Pts',(-0.522570642853263,-0.856100438654279,
-1.63921909308229));
#45413=CARTESIAN_POINT('Ctrl Pts',(-0.646239135575092,-0.749465207577936,
-1.64578685079393));
#45414=CARTESIAN_POINT('Ctrl Pts',(-0.76990762829692,-0.642829976501594,
-1.65235460850557));
#45415=CARTESIAN_POINT('Ctrl Pts',(-0.866620267574799,-0.504933223986081,
-1.65892236621721));
#45416=CARTESIAN_POINT('Ctrl Pts',(-0.924759448763137,-0.352339555833462,
-1.66549012392885));
#45417=CARTESIAN_POINT('Ctrl Pts',(-0.967498363418187,-0.240165843944588,
-1.67031817328517));
#45418=CARTESIAN_POINT('Ctrl Pts',(-0.989392478140921,-0.120050031936858,
-1.67514622264148));
#45419=CARTESIAN_POINT('Ctrl Pts',(-0.989508121607439,2.46417016753209E-5,
-1.67997427199779));
#45420=CARTESIAN_POINT('Ctrl Pts',(-0.989512555708751,1.62595781710845E-5,
-1.71597572800221));
#45421=CARTESIAN_POINT('Ctrl Pts',(-0.989394394624236,-0.121104097426263,
-1.71110554553322));
#45422=CARTESIAN_POINT('Ctrl Pts',(-0.96710644517705,-0.24225952369773,
-1.70623536306422));
#45423=CARTESIAN_POINT('Ctrl Pts',(-0.923634939065364,-0.355272041749406,
-1.70136518059523));
#45424=CARTESIAN_POINT('Ctrl Pts',(-0.865010786619457,-0.507676770252159,
-1.69479742288359));
#45425=CARTESIAN_POINT('Ctrl Pts',(-0.767861633161228,-0.64527258104675,
-1.68822966517194));
#45426=CARTESIAN_POINT('Ctrl Pts',(-0.643855273201409,-0.751516138272709,
-1.6816619074603));
#45427=CARTESIAN_POINT('Ctrl Pts',(-0.519848913241591,-0.857759695498667,
-1.67509414974866));
#45428=CARTESIAN_POINT('Ctrl Pts',(-0.368985346780182,-0.932650999155991,
-1.66852639203702));
#45429=CARTESIAN_POINT('Ctrl Pts',(-0.209388203118329,-0.967201097307302,
-1.66195863432538));
#45430=CARTESIAN_POINT('Ctrl Pts',(-0.0497910594564758,-1.00175119545861,
-1.65539087661374));
#45431=CARTESIAN_POINT('Ctrl Pts',(0.118539661405822,-0.995960088103908,
-1.6488231189021));
#45432=CARTESIAN_POINT('Ctrl Pts',(0.27538380659921,-0.950519709731925,
-1.64225536119046));
#45433=CARTESIAN_POINT('Ctrl Pts',(0.432227951792598,-0.905079331359941,
-1.63568760347881));
#45434=CARTESIAN_POINT('Ctrl Pts',(0.577585521317075,-0.819989681970679,
-1.62911984576717));
#45435=CARTESIAN_POINT('Ctrl Pts',(0.693995143032626,-0.705474038967786,
-1.62255208805553));
#45436=CARTESIAN_POINT('Ctrl Pts',(0.810404764748177,-0.590958395964892,
-1.61598433034389));
#45437=CARTESIAN_POINT('Ctrl Pts',(0.897866438654801,-0.447016759348368,
-1.60941657263225));
#45438=CARTESIAN_POINT('Ctrl Pts',(0.945873977571743,-0.290939168622987,
-1.60284881492061));
#45439=CARTESIAN_POINT('Ctrl Pts',(0.993881516488684,-0.134861577897606,
-1.59628105720897));
#45440=CARTESIAN_POINT('Ctrl Pts',(1.00243492041594,0.0333519669366303,
-1.58971329949732));
#45441=CARTESIAN_POINT('Ctrl Pts',(0.970506636916252,0.193494330149772,
-1.58314554178568));
#45442=CARTESIAN_POINT('Ctrl Pts',(0.938578353416562,0.353636693362912,
-1.57657778407404));
#45443=CARTESIAN_POINT('Ctrl Pts',(0.866168382489923,0.505707874954959,
-1.5700100263624));
#45444=CARTESIAN_POINT('Ctrl Pts',(0.761975010695729,0.631440565385368,
-1.56344226865076));
#45445=CARTESIAN_POINT('Ctrl Pts',(0.657781638901535,0.757173255815777,
-1.55687451093912));
#45446=CARTESIAN_POINT('Ctrl Pts',(0.521804866239785,0.856567455084549,
-1.55030675322748));
#45447=CARTESIAN_POINT('Ctrl Pts',(0.370378885396273,0.917683310519167,
-1.54373899551583));
#45448=CARTESIAN_POINT('Ctrl Pts',(0.218952904552762,0.978799165953784,
-1.53717123780419));
#45449=CARTESIAN_POINT('Ctrl Pts',(0.0520777155274912,1.00163667755425,
-1.53060348009255));
#45450=CARTESIAN_POINT('Ctrl Pts',(-0.110200787535187,0.983452551133096,
-1.52403572238091));
#45451=CARTESIAN_POINT('Ctrl Pts',(-0.272479290597865,0.965268424711947,
-1.51746796466927));
#45452=CARTESIAN_POINT('Ctrl Pts',(-0.430161107697951,0.906062660269186,
-1.51090020695763));
#45453=CARTESIAN_POINT('Ctrl Pts',(-0.564304713162749,0.812947319648577,
-1.50433244924599));
#45454=CARTESIAN_POINT('Ctrl Pts',(-0.698448318627548,0.719831979027969,
-1.49776469153435));
#45455=CARTESIAN_POINT('Ctrl Pts',(-0.809053712457058,0.592807062229512,
-1.4911969338227));
#45456=CARTESIAN_POINT('Ctrl Pts',(-0.88283441765268,0.447131455127287,
-1.48462917611106));
#45457=CARTESIAN_POINT('Ctrl Pts',(-0.952683957187391,0.309217700432873,
-1.47841136007478));
#45458=CARTESIAN_POINT('Ctrl Pts',(-0.989528433074503,0.154587790262781,
-1.47219354403849));
#45459=CARTESIAN_POINT('Ctrl Pts',(-0.989600974548901,-8.74702472718336E-6,
-1.46597572800221));
#45460=CARTESIAN_POINT('Origin',(0.,0.,-0.915));
#45461=CARTESIAN_POINT('',(-0.989468413969488,-1.8577996640623E-5,-1.17997427199779));
#45462=CARTESIAN_POINT('',(-0.989466234208983,-1.79285505235583E-5,-1.21597572800221));
#45463=CARTESIAN_POINT('',(-0.989525,-1.21181862392628E-16,-0.915));
#45464=CARTESIAN_POINT('Ctrl Pts',(-0.989468413969488,-1.8577996640623E-5,
-1.17997427199779));
#45465=CARTESIAN_POINT('Ctrl Pts',(-0.989396562633886,0.104757608424716,
-1.18418670422875));
#45466=CARTESIAN_POINT('Ctrl Pts',(-0.972819916344485,0.209555998775421,
-1.18839913645971));
#45467=CARTESIAN_POINT('Ctrl Pts',(-0.940111910177114,0.309051383145319,
-1.19261156869068));
#45468=CARTESIAN_POINT('Ctrl Pts',(-0.889115657190716,0.464178288965946,
-1.19917932640232));
#45469=CARTESIAN_POINT('Ctrl Pts',(-0.798905564248481,0.606414079010267,
-1.20574708411396));
#45470=CARTESIAN_POINT('Ctrl Pts',(-0.680318120066929,0.718672676946543,
-1.2123148418256));
#45471=CARTESIAN_POINT('Ctrl Pts',(-0.561730675885377,0.830931274882821,
-1.21888259953724));
#45472=CARTESIAN_POINT('Ctrl Pts',(-0.414765880464508,0.913212680711054,
-1.22545035724888));
#45473=CARTESIAN_POINT('Ctrl Pts',(-0.257077881975125,0.955632839368786,
-1.23201811496052));
#45474=CARTESIAN_POINT('Ctrl Pts',(-0.0993898834857447,0.998052998026518,
-1.23858587267216));
#45475=CARTESIAN_POINT('Ctrl Pts',(0.0690213180721501,1.00061190951375,
-1.24515363038381));
#45476=CARTESIAN_POINT('Ctrl Pts',(0.227925324681052,0.963002184551002,
-1.25172138809545));
#45477=CARTESIAN_POINT('Ctrl Pts',(0.386829331289954,0.925392459588256,
-1.25828914580709));
#45478=CARTESIAN_POINT('Ctrl Pts',(0.536226142949864,0.847614098175531,
-1.26485690351873));
#45479=CARTESIAN_POINT('Ctrl Pts',(0.658169465504165,0.73901022710025,-1.27142466123037));
#45480=CARTESIAN_POINT('Ctrl Pts',(0.780112788058465,0.630406356024968,
-1.27799241894201));
#45481=CARTESIAN_POINT('Ctrl Pts',(0.874602621507156,0.490976975287128,
-1.28456017665365));
#45482=CARTESIAN_POINT('Ctrl Pts',(0.930288373243623,0.337471041259424,
-1.2911279343653));
#45483=CARTESIAN_POINT('Ctrl Pts',(0.98597412498009,0.18396510723172,-1.29769569207694));
#45484=CARTESIAN_POINT('Ctrl Pts',(1.00285579500433,0.0163826199141512,
-1.30426344978858));
#45485=CARTESIAN_POINT('Ctrl Pts',(0.978905472461058,-0.145145571984733,
-1.31083120750022));
#45486=CARTESIAN_POINT('Ctrl Pts',(0.954955149917781,-0.306673763883617,
-1.31739896521186));
#45487=CARTESIAN_POINT('Ctrl Pts',(0.890172834806985,-0.462147660363816,
-1.3239667229235));
#45488=CARTESIAN_POINT('Ctrl Pts',(0.79234050366626,-0.592890957369197,
-1.33053448063514));
#45489=CARTESIAN_POINT('Ctrl Pts',(0.694508172525535,-0.723634254374579,
-1.33710223834679));
#45490=CARTESIAN_POINT('Ctrl Pts',(0.563625825354881,-0.829646951905141,
-1.34366999605843));
#45491=CARTESIAN_POINT('Ctrl Pts',(0.415415705996909,-0.898194273135755,
-1.35023775377007));
#45492=CARTESIAN_POINT('Ctrl Pts',(0.267205586638937,-0.966741594366368,
-1.35680551148171));
#45493=CARTESIAN_POINT('Ctrl Pts',(0.101667695093648,-0.997823539297033,
-1.36337326919335));
#45494=CARTESIAN_POINT('Ctrl Pts',(-0.0613127270280904,-0.98770638885309,
-1.36994102690499));
#45495=CARTESIAN_POINT('Ctrl Pts',(-0.224293149149829,-0.977589238409147,
-1.37650878461663));
#45496=CARTESIAN_POINT('Ctrl Pts',(-0.384716101848015,-0.926272992590596,
-1.38307654232827));
#45497=CARTESIAN_POINT('Ctrl Pts',(-0.523310775614874,-0.839922016149752,
-1.38964430003991));
#45498=CARTESIAN_POINT('Ctrl Pts',(-0.661905449381735,-0.753571039708906,
-1.39621205775156));
#45499=CARTESIAN_POINT('Ctrl Pts',(-0.778671844217267,-0.632185332645765,
-1.4027798154632));
#45500=CARTESIAN_POINT('Ctrl Pts',(-0.859583395256424,-0.490346354807054,
-1.40934757317484));
#45501=CARTESIAN_POINT('Ctrl Pts',(-0.940494946295581,-0.348507376968345,
-1.41591533088648));
#45502=CARTESIAN_POINT('Ctrl Pts',(-0.985551653538363,-0.186215128354065,
-1.42248308859812));
#45503=CARTESIAN_POINT('Ctrl Pts',(-0.989341079377716,-0.0229649676037106,
-1.42905084630976));
#45504=CARTESIAN_POINT('Ctrl Pts',(-0.989518676934171,-0.0153139854050142,
-1.42935865487244));
#45505=CARTESIAN_POINT('Ctrl Pts',(-0.989605631754353,-0.00766089917197932,
-1.42966646343512));
#45506=CARTESIAN_POINT('Ctrl Pts',(-0.989602407284016,-7.73947795529306E-6,
-1.42997427199779));
#45507=CARTESIAN_POINT('Ctrl Pts',(-0.989600974548901,-8.74702472718336E-6,
-1.46597572800221));
#45508=CARTESIAN_POINT('Ctrl Pts',(-0.989605057217949,-0.00870951445610583,
-1.46562578632685));
#45509=CARTESIAN_POINT('Ctrl Pts',(-0.989492665060294,-0.017410176179129,
-1.4652758446515));
#45510=CARTESIAN_POINT('Ctrl Pts',(-0.989263126563413,-0.026107746288861,
-1.46492590297614));
#45511=CARTESIAN_POINT('Ctrl Pts',(-0.984955113716792,-0.18934504319679,
-1.4583581452645));
#45512=CARTESIAN_POINT('Ctrl Pts',(-0.939383071461817,-0.351493339606654,
-1.45179038755286));
#45513=CARTESIAN_POINT('Ctrl Pts',(-0.858021341400782,-0.493074565003882,
-1.44522262984121));
#45514=CARTESIAN_POINT('Ctrl Pts',(-0.776659611339746,-0.634655790401111,
-1.43865487212957));
#45515=CARTESIAN_POINT('Ctrl Pts',(-0.659508193472649,-0.755669944785702,
-1.43208711441793));
#45516=CARTESIAN_POINT('Ctrl Pts',(-0.520639903880605,-0.841580203173077,
-1.42551935670629));
#45517=CARTESIAN_POINT('Ctrl Pts',(-0.38177161428856,-0.927490461560451,
-1.41895159899465));
#45518=CARTESIAN_POINT('Ctrl Pts',(-0.221186452971569,-0.97829682395061,
-1.41238384128301));
#45519=CARTESIAN_POINT('Ctrl Pts',(-0.0581747145888518,-0.987896174287954,
-1.40581608357137));
#45520=CARTESIAN_POINT('Ctrl Pts',(0.104837023793865,-0.997495524625299,
-1.39924832585972));
#45521=CARTESIAN_POINT('Ctrl Pts',(0.270275339242308,-0.96588786290983,
-1.39268056814808));
#45522=CARTESIAN_POINT('Ctrl Pts',(0.418266951644149,-0.896870060487294,
-1.38611281043644));
#45523=CARTESIAN_POINT('Ctrl Pts',(0.566258564045989,-0.827852258064758,
-1.3795450527248));
#45524=CARTESIAN_POINT('Ctrl Pts',(0.696803473401228,-0.721424314935155,
-1.37297729501316));
#45525=CARTESIAN_POINT('Ctrl Pts',(0.794219970630926,-0.590370889036802,
-1.36640953730152));
#45526=CARTESIAN_POINT('Ctrl Pts',(0.891636467860624,-0.45931746313845,
-1.35984177958988));
#45527=CARTESIAN_POINT('Ctrl Pts',(0.955924552964781,-0.303638554471347,
-1.35327402187823));
#45528=CARTESIAN_POINT('Ctrl Pts',(0.979361618771641,-0.142035094320265,
-1.34670626416659));
#45529=CARTESIAN_POINT('Ctrl Pts',(1.0027986845785,0.0195683658308168,-1.34013850645495));
#45530=CARTESIAN_POINT('Ctrl Pts',(0.985384731088064,0.18709637746588,-1.33357074874331));
#45531=CARTESIAN_POINT('Ctrl Pts',(0.929211609725224,0.340424635837656,
-1.32700299103167));
#45532=CARTESIAN_POINT('Ctrl Pts',(0.873038488362384,0.493752894209432,
-1.32043523332003));
#45533=CARTESIAN_POINT('Ctrl Pts',(0.778106199127141,0.632881399317924,
-1.31386747560839));
#45534=CARTESIAN_POINT('Ctrl Pts',(0.655818484628525,0.741097337444794,
-1.30729971789675));
#45535=CARTESIAN_POINT('Ctrl Pts',(0.533530770129908,0.849313275571664,
-1.3007319601851));
#45536=CARTESIAN_POINT('Ctrl Pts',(0.383887630367918,0.926616646716914,
-1.29416420247346));
#45537=CARTESIAN_POINT('Ctrl Pts',(0.224864949668683,0.963721382323536,
-1.28759644476182));
#45538=CARTESIAN_POINT('Ctrl Pts',(0.065842268969448,1.00082611793016,-1.28102868705018));
#45539=CARTESIAN_POINT('Ctrl Pts',(-0.102559952667031,0.997732217998152,
-1.27446092933854));
#45540=CARTESIAN_POINT('Ctrl Pts',(-0.260112395937802,0.954811337292705,
-1.2678931716269));
#45541=CARTESIAN_POINT('Ctrl Pts',(-0.417664839208572,0.911890456587258,
-1.26132541391526));
#45542=CARTESIAN_POINT('Ctrl Pts',(-0.564367504113633,0.829142595108368,
-1.25475765620361));
#45543=CARTESIAN_POINT('Ctrl Pts',(-0.682597730913487,0.716507840914783,
-1.24818989849197));
#45544=CARTESIAN_POINT('Ctrl Pts',(-0.80082795771334,0.603873086721197,
-1.24162214078033));
#45545=CARTESIAN_POINT('Ctrl Pts',(-0.890585746407986,0.461351439812916,
-1.23505438306869));
#45546=CARTESIAN_POINT('Ctrl Pts',(-0.941088941335523,0.306063315079296,
-1.22848662535705));
#45547=CARTESIAN_POINT('Ctrl Pts',(-0.973156724363405,0.207460723740084,
-1.22431632623877));
#45548=CARTESIAN_POINT('Ctrl Pts',(-0.98939779705991,0.103710929816322,
-1.22014602712049));
#45549=CARTESIAN_POINT('Ctrl Pts',(-0.989466234208983,-1.79285505235583E-5,
-1.21597572800221));
#45550=CARTESIAN_POINT('Origin',(0.,0.,-0.915));
#45551=CARTESIAN_POINT('',(-0.989479227929023,2.11592729404686E-5,-0.929974271997791));
#45552=CARTESIAN_POINT('',(-0.989481817826863,2.16465008535149E-5,-0.965975728002209));
#45553=CARTESIAN_POINT('',(-0.989525,-1.21181862392628E-16,-0.915));
#45554=CARTESIAN_POINT('Ctrl Pts',(-0.989479227929023,2.11592729404686E-5,
-0.929974271997791));
#45555=CARTESIAN_POINT('Ctrl Pts',(-0.989521950655237,0.0538675948649017,
-0.932139187310748));
#45556=CARTESIAN_POINT('Ctrl Pts',(-0.985200273850893,0.107707242346304,
-0.934304102623705));
#45557=CARTESIAN_POINT('Ctrl Pts',(-0.976453133180159,0.160818033141656,
-0.936469017936662));
#45558=CARTESIAN_POINT('Ctrl Pts',(-0.949916713833314,0.321941567041523,
-0.943036775648303));
#45559=CARTESIAN_POINT('Ctrl Pts',(-0.882650593613209,0.476357077624845,
-0.949604533359944));
#45560=CARTESIAN_POINT('Ctrl Pts',(-0.782735116182012,0.605515399454408,
-0.956172291071585));
#45561=CARTESIAN_POINT('Ctrl Pts',(-0.682819638750815,0.734673721283971,
-0.962740048783226));
#45562=CARTESIAN_POINT('Ctrl Pts',(-0.550254804108526,0.838574854359776,
-0.969307806494868));
#45563=CARTESIAN_POINT('Ctrl Pts',(-0.400964964929612,0.904737673571679,
-0.97587556420651));
#45564=CARTESIAN_POINT('Ctrl Pts',(-0.251675125750698,0.970900492783582,
-0.982443321918151));
#45565=CARTESIAN_POINT('Ctrl Pts',(-0.0856602820351579,0.999324998131584,
-0.989011079629792));
#45566=CARTESIAN_POINT('Ctrl Pts',(0.0771370307198936,0.986596695500557,
-0.995578837341433));
#45567=CARTESIAN_POINT('Ctrl Pts',(0.239934343474945,0.973868392869529,
-1.00214659505307));
#45568=CARTESIAN_POINT('Ctrl Pts',(0.399514125269508,0.919987282259473,
-1.00871435276472));
#45569=CARTESIAN_POINT('Ctrl Pts',(0.536706852512593,0.831425832859988,
-1.01528211047636));
#45570=CARTESIAN_POINT('Ctrl Pts',(0.673899579755678,0.742864383460502,
-1.021849868188));
#45571=CARTESIAN_POINT('Ctrl Pts',(0.788705252447284,0.619622595271587,
-1.02841762589964));
#45572=CARTESIAN_POINT('Ctrl Pts',(0.867332837498556,0.476504889877957,
-1.03498538361128));
#45573=CARTESIAN_POINT('Ctrl Pts',(0.945960422549827,0.333387184484326,
-1.04155314132292));
#45574=CARTESIAN_POINT('Ctrl Pts',(0.988409919960763,0.170393561885978,
-1.04812089903456));
#45575=CARTESIAN_POINT('Ctrl Pts',(0.98958208324228,0.0071036333497253,
-1.05468865674621));
#45576=CARTESIAN_POINT('Ctrl Pts',(0.990754246523798,-0.156186295186527,
-1.06125641445785));
#45577=CARTESIAN_POINT('Ctrl Pts',(0.950649075675897,-0.319772529660686,
-1.06782417216949));
#45578=CARTESIAN_POINT('Ctrl Pts',(0.874084204925446,-0.464004271295804,
-1.07439192988113));
#45579=CARTESIAN_POINT('Ctrl Pts',(0.797519334174994,-0.608236012930923,
-1.08095968759277));
#45580=CARTESIAN_POINT('Ctrl Pts',(0.684494763521991,-0.733113261727003,
-1.08752744530441));
#45581=CARTESIAN_POINT('Ctrl Pts',(0.548587571147204,-0.823635136370293,
-1.09409520301605));
#45582=CARTESIAN_POINT('Ctrl Pts',(0.412680378772416,-0.914157011013583,
-1.1006629607277));
#45583=CARTESIAN_POINT('Ctrl Pts',(0.253890564675843,-0.970323511504083,
-1.10723071843934));
#45584=CARTESIAN_POINT('Ctrl Pts',(0.091292757567354,-0.985387636159825,
-1.11379847615098));
#45585=CARTESIAN_POINT('Ctrl Pts',(-0.0713050495411349,-1.00045176081557,
-1.12036623386262));
#45586=CARTESIAN_POINT('Ctrl Pts',(-0.23771084966154,-0.97441350963655,
-1.12693399157426));
#45587=CARTESIAN_POINT('Ctrl Pts',(-0.38793514365297,-0.910400727921418,
-1.1335017492859));
#45588=CARTESIAN_POINT('Ctrl Pts',(-0.538159437644401,-0.846387946206286,
-1.14006950699754));
#45589=CARTESIAN_POINT('Ctrl Pts',(-0.672202225506858,-0.744400633955038,
-1.14663726470919));
#45590=CARTESIAN_POINT('Ctrl Pts',(-0.773961615413973,-0.616690018523645,
-1.15320502242083));
#45591=CARTESIAN_POINT('Ctrl Pts',(-0.875721005321089,-0.488979403092252,
-1.15977278013247));
#45592=CARTESIAN_POINT('Ctrl Pts',(-0.945196997272862,-0.335545484480712,
-1.16634053784411));
#45593=CARTESIAN_POINT('Ctrl Pts',(-0.974043786733467,-0.174819514376474,
-1.17290829555575));
#45594=CARTESIAN_POINT('Ctrl Pts',(-0.984388805724034,-0.117180059723252,
-1.17526362103643));
#45595=CARTESIAN_POINT('Ctrl Pts',(-0.989508588688577,-0.0586027897099681,
-1.17761894651711));
#45596=CARTESIAN_POINT('Ctrl Pts',(-0.989468413969488,-1.8577996640623E-5,
-1.17997427199779));
#45597=CARTESIAN_POINT('Ctrl Pts',(-0.989466234208983,-1.79285505235583E-5,
-1.21597572800221));
#45598=CARTESIAN_POINT('Ctrl Pts',(-0.989505577965029,-0.0596504958599335,
-1.21357826940885));
#45599=CARTESIAN_POINT('Ctrl Pts',(-0.984199910544476,-0.119276144025869,
-1.21118081081549));
#45600=CARTESIAN_POINT('Ctrl Pts',(-0.973483506439899,-0.177912931038826,
-1.20878335222212));
#45601=CARTESIAN_POINT('Ctrl Pts',(-0.944126275456312,-0.338546449864369,
-1.20221559451048));
#45602=CARTESIAN_POINT('Ctrl Pts',(-0.874163212328713,-0.491758884956497,
-1.19564783679884));
#45603=CARTESIAN_POINT('Ctrl Pts',(-0.771998631025041,-0.619145590339313,
-1.1890800790872));
#45604=CARTESIAN_POINT('Ctrl Pts',(-0.669834049721368,-0.746532295722131,
-1.18251232137556));
#45605=CARTESIAN_POINT('Ctrl Pts',(-0.535467950241621,-0.848093271395637,
-1.17594456366392));
#45606=CARTESIAN_POINT('Ctrl Pts',(-0.385041062224816,-0.911628503691119,
-1.16937680595228));
#45607=CARTESIAN_POINT('Ctrl Pts',(-0.234614174208011,-0.975163735986602,
-1.16280904824063));
#45608=CARTESIAN_POINT('Ctrl Pts',(-0.0681264976541487,-1.00067322490406,
-1.15624129052899));
#45609=CARTESIAN_POINT('Ctrl Pts',(0.0944226328881091,-0.985092642719303,
-1.14967353281735));
#45610=CARTESIAN_POINT('Ctrl Pts',(0.256971763430366,-0.969512060534544,
-1.14310577510571));
#45611=CARTESIAN_POINT('Ctrl Pts',(0.415582347961017,-0.912841407247569,
-1.13653801739407));
#45612=CARTESIAN_POINT('Ctrl Pts',(0.551201287724399,-0.821888245902224,
-1.12997025968243));
#45613=CARTESIAN_POINT('Ctrl Pts',(0.686820227487781,-0.730935084556877,
-1.12340250197079));
#45614=CARTESIAN_POINT('Ctrl Pts',(0.799447522483893,-0.60569941515316,
-1.11683474425915));
#45615=CARTESIAN_POINT('Ctrl Pts',(0.875553817275981,-0.461225174285523,
-1.1102669865475));
#45616=CARTESIAN_POINT('Ctrl Pts',(0.951660112068069,-0.316750933417886,
-1.10369922883586));
#45617=CARTESIAN_POINT('Ctrl Pts',(0.991245406656133,-0.153038121086327,
-1.09713147112422));
#45618=CARTESIAN_POINT('Ctrl Pts',(0.989554516956521,0.0102472587652755,
-1.09056371341258));
#45619=CARTESIAN_POINT('Ctrl Pts',(0.987863627256909,0.173532638616877,
-1.08399595570094));
#45620=CARTESIAN_POINT('Ctrl Pts',(0.944896553269623,0.336390585988523,
-1.0774281979893));
#45621=CARTESIAN_POINT('Ctrl Pts',(0.865814715377448,0.479257787601961,
-1.07086044027766));
#45622=CARTESIAN_POINT('Ctrl Pts',(0.786732877485274,0.622124989215399,
-1.06429268256602));
#45623=CARTESIAN_POINT('Ctrl Pts',(0.67153627568821,0.745001445070627,-1.05772492485437));
#45624=CARTESIAN_POINT('Ctrl Pts',(0.53406290343955,0.833126619134794,-1.05115716714273));
#45625=CARTESIAN_POINT('Ctrl Pts',(0.39658953119089,0.921251793198961,-1.04458940943109));
#45626=CARTESIAN_POINT('Ctrl Pts',(0.236839388490635,0.974625685472067,
-1.03802165171945));
#45627=CARTESIAN_POINT('Ctrl Pts',(0.0740024635360275,0.986836756374557,
-1.03145389400781));
#45628=CARTESIAN_POINT('Ctrl Pts',(-0.0888344614185813,0.999047827277046,
-1.02488613629617));
#45629=CARTESIAN_POINT('Ctrl Pts',(-0.254758168627542,0.970096076808919,
-1.01831837858452));
#45630=CARTESIAN_POINT('Ctrl Pts',(-0.403837070367909,0.903459334412967,
-1.01175062087288));
#45631=CARTESIAN_POINT('Ctrl Pts',(-0.552915972108275,0.836822592017015,
-1.00518286316124));
#45632=CARTESIAN_POINT('Ctrl Pts',(-0.685150068380046,0.73250085769324,
-0.998615105449601));
#45633=CARTESIAN_POINT('Ctrl Pts',(-0.78465473646029,0.603025781282765,
-0.99204734773796));
#45634=CARTESIAN_POINT('Ctrl Pts',(-0.884159404540536,0.473550704872287,
-0.985479590026318));
#45635=CARTESIAN_POINT('Ctrl Pts',(-0.950934644429253,0.318922286375109,
-0.978911832314676));
#45636=CARTESIAN_POINT('Ctrl Pts',(-0.976959079471164,0.157715266794669,
-0.972344074603035));
#45637=CARTESIAN_POINT('Ctrl Pts',(-0.985370505395306,0.105611123074779,
-0.97022129240276));
#45638=CARTESIAN_POINT('Ctrl Pts',(-0.989524841441287,0.0528197365828913,
-0.968098510202484));
#45639=CARTESIAN_POINT('Ctrl Pts',(-0.989481817826863,2.16465008535149E-5,
-0.965975728002209));
#45640=CARTESIAN_POINT('Origin',(0.,0.,-0.915));
#45641=CARTESIAN_POINT('',(-0.989606782241323,3.0037068674809E-6,-0.67997427199779));
#45642=CARTESIAN_POINT('',(-0.989607241147724,1.92919255151051E-6,-0.71597572800221));
#45643=CARTESIAN_POINT('',(-0.989525,-1.21181862392628E-16,-0.915));
#45644=CARTESIAN_POINT('Ctrl Pts',(-0.989606782241323,3.0037068674809E-6,
-0.67997427199779));
#45645=CARTESIAN_POINT('Ctrl Pts',(-0.989607295470647,0.00292188642515435,
-0.680091670392743));
#45646=CARTESIAN_POINT('Ctrl Pts',(-0.989594647512363,0.00584076467806051,
-0.680209068787695));
#45647=CARTESIAN_POINT('Ctrl Pts',(-0.989568811039347,0.00875952618805917,
-0.680326467182648));
#45648=CARTESIAN_POINT('Ctrl Pts',(-0.988123410572325,0.172047264691672,
-0.686894224894289));
#45649=CARTESIAN_POINT('Ctrl Pts',(-0.945401229584537,0.334969626845597,
-0.69346198260593));
#45650=CARTESIAN_POINT('Ctrl Pts',(-0.8665342706836,0.477955561544956,-0.700029740317572));
#45651=CARTESIAN_POINT('Ctrl Pts',(-0.787667311782663,0.620941496244314,
-0.706597498029213));
#45652=CARTESIAN_POINT('Ctrl Pts',(-0.672655574968577,0.743991003489105,
-0.713165255740855));
#45653=CARTESIAN_POINT('Ctrl Pts',(-0.535314846785921,0.832322759445795,
-0.719733013452496));
#45654=CARTESIAN_POINT('Ctrl Pts',(-0.397974118603265,0.920654515402485,
-0.726300771164138));
#45655=CARTESIAN_POINT('Ctrl Pts',(-0.238304399052039,0.974268520071073,
-0.732868528875779));
#45656=CARTESIAN_POINT('Ctrl Pts',(-0.0754860154975323,0.986724390367039,
-0.73943628658742));
#45657=CARTESIAN_POINT('Ctrl Pts',(0.0873323680569721,0.999180260663004,
-0.746004044299061));
#45658=CARTESIAN_POINT('Ctrl Pts',(0.253299415614757,0.970477996586349,
-0.752571802010703));
#45659=CARTESIAN_POINT('Ctrl Pts',(0.40247833319284,0.904065458023485,-0.759139559722344));
#45660=CARTESIAN_POINT('Ctrl Pts',(0.551657250770926,0.837652919460619,
-0.765707317433986));
#45661=CARTESIAN_POINT('Ctrl Pts',(0.68404803836931,0.733530106411544,-0.772275075145627));
#45662=CARTESIAN_POINT('Ctrl Pts',(0.78374725071719,0.604204773296391,-0.778842832857268));
#45663=CARTESIAN_POINT('Ctrl Pts',(0.88344646306507,0.47487944018124,-0.78541059056891));
#45664=CARTESIAN_POINT('Ctrl Pts',(0.950454100162448,0.320351587000007,
-0.791978348280551));
#45665=CARTESIAN_POINT('Ctrl Pts',(0.976720868636,0.159183874346109,-0.798546105992192));
#45666=CARTESIAN_POINT('Ctrl Pts',(1.00298763710955,-0.00198383830779042,
-0.805113863703834));
#45667=CARTESIAN_POINT('Ctrl Pts',(0.988513536959279,-0.169791410434359,
-0.811681621415475));
#45668=CARTESIAN_POINT('Ctrl Pts',(0.935037269674611,-0.324080955010237,
-0.818249379127116));
#45669=CARTESIAN_POINT('Ctrl Pts',(0.881561002389944,-0.478370499586115,
-0.824817136838758));
#45670=CARTESIAN_POINT('Ctrl Pts',(0.789082567970882,-0.619142016611303,
-0.831384894550399));
#45671=CARTESIAN_POINT('Ctrl Pts',(0.668710939686584,-0.729485325571656,
-0.837952652262041));
#45672=CARTESIAN_POINT('Ctrl Pts',(0.548339311402286,-0.839828634532009,
-0.844520409973682));
#45673=CARTESIAN_POINT('Ctrl Pts',(0.400074489252753,-0.919743735427527,
-0.851088167685324));
#45674=CARTESIAN_POINT('Ctrl Pts',(0.241726787138328,-0.95963082560987,
-0.857655925396965));
#45675=CARTESIAN_POINT('Ctrl Pts',(0.0833790850239023,-0.999517915792213,
-0.864223683108606));
#45676=CARTESIAN_POINT('Ctrl Pts',(-0.0850514970554142,-0.99937699526138,
-0.870791440820247));
#45677=CARTESIAN_POINT('Ctrl Pts',(-0.243332232996699,-0.959224992098172,
-0.877359198531889));
#45678=CARTESIAN_POINT('Ctrl Pts',(-0.401612968937987,-0.919072988934964,
-0.88392695624353));
#45679=CARTESIAN_POINT('Ctrl Pts',(-0.549743858741242,-0.838909903139379,
-0.890494713955172));
#45680=CARTESIAN_POINT('Ctrl Pts',(-0.66993067713115,-0.728365326549457,
-0.897062471666814));
#45681=CARTESIAN_POINT('Ctrl Pts',(-0.790117495521055,-0.617820749959539,
-0.903630229378455));
#45682=CARTESIAN_POINT('Ctrl Pts',(-0.882360242497614,-0.476894682575286,
-0.910197987090096));
#45683=CARTESIAN_POINT('Ctrl Pts',(-0.935578256749101,-0.322515870274955,
-0.916765744801737));
#45684=CARTESIAN_POINT('Ctrl Pts',(-0.971254135764085,-0.219024601245696,
-0.921168587200421));
#45685=CARTESIAN_POINT('Ctrl Pts',(-0.989392341652577,-0.109487683046862,
-0.925571429599106));
#45686=CARTESIAN_POINT('Ctrl Pts',(-0.989479227929023,2.11592729404686E-5,
-0.929974271997791));
#45687=CARTESIAN_POINT('Ctrl Pts',(-0.989481817826863,2.16465008535149E-5,
-0.965975728002209));
#45688=CARTESIAN_POINT('Ctrl Pts',(-0.989391729021473,-0.110534310408492,
-0.961530752490843));
#45689=CARTESIAN_POINT('Ctrl Pts',(-0.970897986417988,-0.221119659736481,
-0.957085776979477));
#45690=CARTESIAN_POINT('Ctrl Pts',(-0.934548975441814,-0.325486345092866,
-0.952640801468111));
#45691=CARTESIAN_POINT('Ctrl Pts',(-0.880840806175447,-0.479695316736262,
-0.94607304375647));
#45692=CARTESIAN_POINT('Ctrl Pts',(-0.788150837447608,-0.620327639359355,
-0.939505286044829));
#45693=CARTESIAN_POINT('Ctrl Pts',(-0.667613453089349,-0.73048985317756,
-0.932937528333187));
#45694=CARTESIAN_POINT('Ctrl Pts',(-0.547076068731089,-0.840652066995765,
-0.926369770621545));
#45695=CARTESIAN_POINT('Ctrl Pts',(-0.398691268742412,-0.920344172009081,
-0.919802012909904));
#45696=CARTESIAN_POINT('Ctrl Pts',(-0.240283779363316,-0.959993152952737,
-0.913234255198263));
#45697=CARTESIAN_POINT('Ctrl Pts',(-0.0818762899842206,-0.999642133896393,
-0.906666497486621));
#45698=CARTESIAN_POINT('Ctrl Pts',(0.0865538887852915,-0.999247990770388,
-0.90009873977498));
#45699=CARTESIAN_POINT('Ctrl Pts',(0.244774079289893,-0.958858070023422,
-0.893530982063339));
#45700=CARTESIAN_POINT('Ctrl Pts',(0.402994269794494,-0.918468149276455,
-0.886963224351698));
#45701=CARTESIAN_POINT('Ctrl Pts',(0.551004472034184,-0.838082450908528,
-0.880395466640056));
#45702=CARTESIAN_POINT('Ctrl Pts',(0.671024958328965,-0.727357308096143,
-0.873827708928415));
#45703=CARTESIAN_POINT('Ctrl Pts',(0.791045444623745,-0.616632165283759,
-0.867259951216773));
#45704=CARTESIAN_POINT('Ctrl Pts',(0.883076214973616,-0.475567578026917,
-0.860692193505132));
#45705=CARTESIAN_POINT('Ctrl Pts',(0.936062071762188,-0.32110893190557,
-0.854124435793491));
#45706=CARTESIAN_POINT('Ctrl Pts',(0.989047928550761,-0.166650285784224,
-0.84755667808185));
#45707=CARTESIAN_POINT('Ctrl Pts',(1.00298887177804,0.00120241920163183,
-0.840988920370208));
#45708=CARTESIAN_POINT('Ctrl Pts',(0.976210245437653,0.162285874443257,
-0.834421162658567));
#45709=CARTESIAN_POINT('Ctrl Pts',(0.94943161909727,0.323369329684882,-0.827853404946925));
#45710=CARTESIAN_POINT('Ctrl Pts',(0.881933423189232,0.477683535182278,
-0.821285647235283));
#45711=CARTESIAN_POINT('Ctrl Pts',(0.781823879471064,0.606691494773144,
-0.814717889523642));
#45712=CARTESIAN_POINT('Ctrl Pts',(0.681714335752896,0.735699454364011,
-0.808150131812001));
#45713=CARTESIAN_POINT('Ctrl Pts',(0.548993444224598,0.839401168048346,
-0.80158237410036));
#45714=CARTESIAN_POINT('Ctrl Pts',(0.399604303896325,0.905339465973283,
-0.795014616388719));
#45715=CARTESIAN_POINT('Ctrl Pts',(0.250215163568049,0.971277763898222,
-0.788446858677077));
#45716=CARTESIAN_POINT('Ctrl Pts',(0.0841577744397947,0.999452646063762,
-0.781879100965435));
#45717=CARTESIAN_POINT('Ctrl Pts',(-0.078620217223007,0.986479604343173,
-0.775311343253794));
#45718=CARTESIAN_POINT('Ctrl Pts',(-0.241398208885805,0.973506562622584,
-0.768743585542152));
#45719=CARTESIAN_POINT('Ctrl Pts',(-0.400896803083149,0.919385597015869,
-0.762175827830512));
#45720=CARTESIAN_POINT('Ctrl Pts',(-0.53795622888534,0.830617989297559,
-0.755608070118871));
#45721=CARTESIAN_POINT('Ctrl Pts',(-0.675015654687532,0.741850381579249,
-0.749040312407229));
#45722=CARTESIAN_POINT('Ctrl Pts',(-0.78963591209457,0.618436131749344,
-0.742472554695587));
#45723=CARTESIAN_POINT('Ctrl Pts',(-0.86804824103133,0.475200378349671,
-0.735904796983945));
#45724=CARTESIAN_POINT('Ctrl Pts',(-0.94646056996809,0.331964624949999,
-0.729337039272304));
#45725=CARTESIAN_POINT('Ctrl Pts',(-0.988664970434574,0.168907367980558,
-0.722769281560663));
#45726=CARTESIAN_POINT('Ctrl Pts',(-0.989591638215686,0.00561586278790557,
-0.716201523849022));
#45727=CARTESIAN_POINT('Ctrl Pts',(-0.989602257656167,0.00374457249822986,
-0.716126258566751));
#45728=CARTESIAN_POINT('Ctrl Pts',(-0.98960745620187,0.00187325144535842,
-0.716050993284481));
#45729=CARTESIAN_POINT('Ctrl Pts',(-0.989607241147724,1.92919255151051E-6,
-0.71597572800221));
#45730=CARTESIAN_POINT('Origin',(0.,0.,-0.915));
#45731=CARTESIAN_POINT('',(-0.98949450850966,-2.34504978581795E-5,-0.429974271997791));
#45732=CARTESIAN_POINT('',(-0.989491623038811,-2.31174877268823E-5,-0.465975728002209));
#45733=CARTESIAN_POINT('',(-0.989525,-1.21181862392628E-16,-0.915));
#45734=CARTESIAN_POINT('Ctrl Pts',(-0.98949450850966,-2.34504978581795E-5,
-0.429974271997791));
#45735=CARTESIAN_POINT('Ctrl Pts',(-0.989390629923838,0.11532021613374,
-0.43461191118638));
#45736=CARTESIAN_POINT('Ctrl Pts',(-0.969224635588088,0.230699262194344,
-0.439249550374969));
#45737=CARTESIAN_POINT('Ctrl Pts',(-0.929722368496541,0.339027253322421,
-0.443887189563558));
#45738=CARTESIAN_POINT('Ctrl Pts',(-0.873779827740854,0.492439791509651,
-0.4504549472752));
#45739=CARTESIAN_POINT('Ctrl Pts',(-0.779056814575157,0.631710863824647,
-0.457022704986841));
#45740=CARTESIAN_POINT('Ctrl Pts',(-0.656931932066817,0.740110530759358,
-0.463590462698482));
#45741=CARTESIAN_POINT('Ctrl Pts',(-0.534807049558477,0.848510197694069,
-0.470158220410124));
#45742=CARTESIAN_POINT('Ctrl Pts',(-0.385280297707493,0.926038459248495,
-0.476725978121765));
#45743=CARTESIAN_POINT('Ctrl Pts',(-0.226313579867206,0.963382231852442,
-0.483293735833407));
#45744=CARTESIAN_POINT('Ctrl Pts',(-0.0673468620269185,1.00072600445639,
-0.489861493545048));
#45745=CARTESIAN_POINT('Ctrl Pts',(0.101059821802673,0.997885288109858,
-0.496429251256689));
#45746=CARTESIAN_POINT('Ctrl Pts',(0.258676616361611,0.955201323921211,
-0.502997008968331));
#45747=CARTESIAN_POINT('Ctrl Pts',(0.41629341092055,0.912517359732565,-0.509564766679972));
#45748=CARTESIAN_POINT('Ctrl Pts',(0.563120316208835,0.829990147701802,
-0.516132524391613));
#45749=CARTESIAN_POINT('Ctrl Pts',(0.681519748076804,0.717533270356876,
-0.522700282103255));
#45750=CARTESIAN_POINT('Ctrl Pts',(0.799919179944774,0.60507639301195,-0.529268039814896));
#45751=CARTESIAN_POINT('Ctrl Pts',(0.889891138392427,0.46268985035286,-0.535835797526538));
#45752=CARTESIAN_POINT('Ctrl Pts',(0.940627740629528,0.307477827875477,
-0.542403555238179));
#45753=CARTESIAN_POINT('Ctrl Pts',(0.991364342866629,0.15226580539809,-0.54897131294982));
#45754=CARTESIAN_POINT('Ctrl Pts',(1.00286558889318,-0.0157716968975903,
-0.555539070661462));
#45755=CARTESIAN_POINT('Ctrl Pts',(0.973749891355825,-0.176449171625418,
-0.562106828373103));
#45756=CARTESIAN_POINT('Ctrl Pts',(0.944634193818474,-0.337126646353242,
-0.568674586084745));
#45757=CARTESIAN_POINT('Ctrl Pts',(0.874901552717228,-0.49044409351321,
-0.575242343796386));
#45758=CARTESIAN_POINT('Ctrl Pts',(0.772928602574952,-0.617984252551632,
-0.581810101508027));
#45759=CARTESIAN_POINT('Ctrl Pts',(0.670955652432676,-0.745524411590054,
-0.588377859219668));
#45760=CARTESIAN_POINT('Ctrl Pts',(0.536742393249371,-0.847287282506928,
-0.594945616931309));
#45761=CARTESIAN_POINT('Ctrl Pts',(0.38641119471913,-0.911048598965344,
-0.601513374642951));
#45762=CARTESIAN_POINT('Ctrl Pts',(0.236079996188885,-0.974809915423762,
-0.608081132354592));
#45763=CARTESIAN_POINT('Ctrl Pts',(0.0696308583117035,-1.00056967742372,
-0.614648890066234));
#45764=CARTESIAN_POINT('Ctrl Pts',(-0.092941513821779,-0.985233493182963,
-0.621216647777876));
#45765=CARTESIAN_POINT('Ctrl Pts',(-0.255513885955259,-0.969897308942204,
-0.627784405489517));
#45766=CARTESIAN_POINT('Ctrl Pts',(-0.414209492345041,-0.91346517846073,
-0.634352163201158));
#45767=CARTESIAN_POINT('Ctrl Pts',(-0.549965020983942,-0.822716012227143,
-0.640919920912799));
#45768=CARTESIAN_POINT('Ctrl Pts',(-0.685720549622844,-0.731966845993555,
-0.647487678624441));
#45769=CARTESIAN_POINT('Ctrl Pts',(-0.798536000510865,-0.606900644007853,
-0.654055436336083));
#45770=CARTESIAN_POINT('Ctrl Pts',(-0.874859415981747,-0.46254098558835,
-0.660623194047724));
#45771=CARTESIAN_POINT('Ctrl Pts',(-0.949818553586881,-0.320761750037418,
-0.667073553364413));
#45772=CARTESIAN_POINT('Ctrl Pts',(-0.989578583273582,-0.160372632977547,
-0.673523912681102));
#45773=CARTESIAN_POINT('Ctrl Pts',(-0.989606782241323,3.0037068674809E-6,
-0.67997427199779));
#45774=CARTESIAN_POINT('Ctrl Pts',(-0.989607241147724,1.92919255151051E-6,
-0.71597572800221));
#45775=CARTESIAN_POINT('Ctrl Pts',(-0.989588690265119,-0.16142104289649,
-0.709483235572839));
#45776=CARTESIAN_POINT('Ctrl Pts',(-0.949287337941748,-0.322852943750881,
-0.702990743143468));
#45777=CARTESIAN_POINT('Ctrl Pts',(-0.873385615756844,-0.465317863970741,
-0.696498250714097));
#45778=CARTESIAN_POINT('Ctrl Pts',(-0.796603990421151,-0.609434332120872,
-0.689930493002456));
#45779=CARTESIAN_POINT('Ctrl Pts',(-0.683391804654025,-0.734141515005271,
-0.683362735290815));
#45780=CARTESIAN_POINT('Ctrl Pts',(-0.547348673904517,-0.82445896048028,
-0.676794977579174));
#45781=CARTESIAN_POINT('Ctrl Pts',(-0.41130554315501,-0.91477640595529,
-0.670227219867532));
#45782=CARTESIAN_POINT('Ctrl Pts',(-0.252431467423123,-0.970704114020911,
-0.66365946215589));
#45783=CARTESIAN_POINT('Ctrl Pts',(-0.0898111973488909,-0.98552376793866,
-0.657091704444249));
#45784=CARTESIAN_POINT('Ctrl Pts',(0.0728090727253406,-1.00034342185641,
-0.650523946732607));
#45785=CARTESIAN_POINT('Ctrl Pts',(0.239175537141915,-0.974055021626288,
-0.643956189020967));
#45786=CARTESIAN_POINT('Ctrl Pts',(0.389303421961953,-0.909816461705308,
-0.637388431309325));
#45787=CARTESIAN_POINT('Ctrl Pts',(0.539431306781992,-0.845577901784329,
-0.630820673597684));
#45788=CARTESIAN_POINT('Ctrl Pts',(0.673320612005493,-0.743389182172492,
-0.624252915886042));
#45789=CARTESIAN_POINT('Ctrl Pts',(0.774887882910271,-0.615525724287871,
-0.617685158174401));
#45790=CARTESIAN_POINT('Ctrl Pts',(0.876455153815049,-0.487662266403251,
-0.61111740046276));
#45791=CARTESIAN_POINT('Ctrl Pts',(0.945700390401103,-0.334124070245847,
-0.604549642751119));
#45792=CARTESIAN_POINT('Ctrl Pts',(0.974305507624321,-0.173354913844795,
-0.597981885039477));
#45793=CARTESIAN_POINT('Ctrl Pts',(1.00291062484754,-0.0125857574437444,
-0.591414127327836));
#45794=CARTESIAN_POINT('Ctrl Pts',(0.990875622707922,0.155414359200951,
-0.584846369616194));
#45795=CARTESIAN_POINT('Ctrl Pts',(0.939646206011021,0.31046441965291,-0.578278611904553));
#45796=CARTESIAN_POINT('Ctrl Pts',(0.88841678931412,0.465514480104868,-0.571710854192912));
#45797=CARTESIAN_POINT('Ctrl Pts',(0.797992958059933,0.607614484364092,
-0.56514309648127));
#45798=CARTESIAN_POINT('Ctrl Pts',(0.679236876283086,0.719694667368287,
-0.558575338769629));
#45799=CARTESIAN_POINT('Ctrl Pts',(0.560480794506238,0.831774850372484,
-0.552007581057988));
#45800=CARTESIAN_POINT('Ctrl Pts',(0.413392462206728,0.913835212121657,
-0.545439823346346));
#45801=CARTESIAN_POINT('Ctrl Pts',(0.255640867424106,0.956018250476421,
-0.538872065634705));
#45802=CARTESIAN_POINT('Ctrl Pts',(0.0978892726414824,0.998201288831184,
-0.532304307923063));
#45803=CARTESIAN_POINT('Ctrl Pts',(-0.0705255846242527,1.00050700379154,
-0.525736550211422));
#45804=CARTESIAN_POINT('Ctrl Pts',(-0.229372867212486,0.962658421314677,
-0.51916879249978));
#45805=CARTESIAN_POINT('Ctrl Pts',(-0.388220149800715,0.924809838837817,
-0.512601034788139));
#45806=CARTESIAN_POINT('Ctrl Pts',(-0.537499857711443,0.846806958923747,
-0.506033277076498));
#45807=CARTESIAN_POINT('Ctrl Pts',(-0.659279763879886,0.738019878647646,
-0.499465519364857));
#45808=CARTESIAN_POINT('Ctrl Pts',(-0.781059670048333,0.629232798371543,
-0.492897761653215));
#45809=CARTESIAN_POINT('Ctrl Pts',(-0.875339774474493,0.489661517733408,
-0.486330003941574));
#45810=CARTESIAN_POINT('Ctrl Pts',(-0.930794678249116,0.336072038834401,
-0.479762246229932));
#45811=CARTESIAN_POINT('Ctrl Pts',(-0.969596862864337,0.228604404602891,
-0.475166740154025));
#45812=CARTESIAN_POINT('Ctrl Pts',(-0.989390621669975,0.114273602193131,
-0.470571234078117));
#45813=CARTESIAN_POINT('Ctrl Pts',(-0.989491623038811,-2.31174877268823E-5,
-0.465975728002209));
#45814=CARTESIAN_POINT('Origin',(0.,0.,-0.915));
#45815=CARTESIAN_POINT('',(-0.989456987247134,1.47486280241971E-5,-0.17997427199779));
#45816=CARTESIAN_POINT('',(-0.989459186063674,1.5401373482473E-5,-0.215975728002209));
#45817=CARTESIAN_POINT('',(-0.989525,-1.21181862392628E-16,-0.915));
#45818=CARTESIAN_POINT('Ctrl Pts',(-0.989456987247134,1.47486280241971E-5,
-0.17997427199779));
#45819=CARTESIAN_POINT('Ctrl Pts',(-0.989491616529124,0.064441050262125,
-0.182564394268375));
#45820=CARTESIAN_POINT('Ctrl Pts',(-0.983293285821839,0.128860829012359,
-0.18515451653896));
#45821=CARTESIAN_POINT('Ctrl Pts',(-0.97079687644072,0.192034862932722,
-0.187744638809545));
#45822=CARTESIAN_POINT('Ctrl Pts',(-0.939109805134186,0.352224886843149,
-0.194312396521186));
#45823=CARTESIAN_POINT('Ctrl Pts',(-0.86692769727473,0.504405089817102,
-0.200880154232828));
#45824=CARTESIAN_POINT('Ctrl Pts',(-0.762923262955385,0.630294367333439,
-0.207447911944469));
#45825=CARTESIAN_POINT('Ctrl Pts',(-0.658918828636039,0.756183644849777,
-0.214015669656111));
#45826=CARTESIAN_POINT('Ctrl Pts',(-0.523092067856803,0.8557819969085,-0.220583427367752));
#45827=CARTESIAN_POINT('Ctrl Pts',(-0.371758245998546,0.917125400129355,
-0.227151185079393));
#45828=CARTESIAN_POINT('Ctrl Pts',(-0.22042442414029,0.97846880335021,-0.233718942791035));
#45829=CARTESIAN_POINT('Ctrl Pts',(-0.0535835412030128,1.0015572577332,
-0.240286700502676));
#45830=CARTESIAN_POINT('Ctrl Pts',(0.108722171403071,0.983617146112767,
-0.246854458214317));
#45831=CARTESIAN_POINT('Ctrl Pts',(0.271027884009149,0.965677034492338,
-0.253422215925958));
#45832=CARTESIAN_POINT('Ctrl Pts',(0.428798426284033,0.906708356868494,
-0.2599899736376));
#45833=CARTESIAN_POINT('Ctrl Pts',(0.563081845971233,0.813794785223099,
-0.266557731349241));
#45834=CARTESIAN_POINT('Ctrl Pts',(0.697365265658436,0.720881213577702,
-0.273125489060882));
#45835=CARTESIAN_POINT('Ctrl Pts',(0.808161562757956,0.594022747910746,
-0.279693246772524));
#45836=CARTESIAN_POINT('Ctrl Pts',(0.882161211042825,0.448458233569121,
-0.286261004484165));
#45837=CARTESIAN_POINT('Ctrl Pts',(0.956160859327694,0.302893719227494,
-0.292828762195807));
#45838=CARTESIAN_POINT('Ctrl Pts',(0.993363858797916,0.138623156211191,
-0.299396519907448));
#45839=CARTESIAN_POINT('Ctrl Pts',(0.989301258947878,-0.0246204367359938,
-0.30596427761909));
#45840=CARTESIAN_POINT('Ctrl Pts',(0.985238659097841,-0.187864029683177,
-0.312532035330731));
#45841=CARTESIAN_POINT('Ctrl Pts',(0.939910459927547,-0.35008065256124,
-0.319099793042372));
#45842=CARTESIAN_POINT('Ctrl Pts',(0.858761681530321,-0.491784038779624,
-0.325667550754014));
#45843=CARTESIAN_POINT('Ctrl Pts',(0.777612903133097,-0.633487424998005,
-0.332235308465655));
#45844=CARTESIAN_POINT('Ctrl Pts',(0.660643545508944,-0.754677574556705,
-0.338803066177296));
#45845=CARTESIAN_POINT('Ctrl Pts',(0.52190456983259,-0.840796515164743,
-0.345370823888938));
#45846=CARTESIAN_POINT('Ctrl Pts',(0.383165594156234,-0.926915455772781,
-0.351938581600579));
#45847=CARTESIAN_POINT('Ctrl Pts',(0.222657000427679,-0.977963187430155,
-0.35850633931222));
#45848=CARTESIAN_POINT('Ctrl Pts',(0.0596598780034666,-0.987807602567975,
-0.365074097023862));
#45849=CARTESIAN_POINT('Ctrl Pts',(-0.103337244420748,-0.997652017705794,
-0.371641854735503));
#45850=CARTESIAN_POINT('Ctrl Pts',(-0.268822895540619,-0.966293116324059,
-0.378209612447145));
#45851=CARTESIAN_POINT('Ctrl Pts',(-0.416918105195915,-0.897497885927143,
-0.384777370158786));
#45852=CARTESIAN_POINT('Ctrl Pts',(-0.565013314851208,-0.828702655530228,
-0.391345127870427));
#45853=CARTESIAN_POINT('Ctrl Pts',(-0.695718083041927,-0.722471096118137,
-0.397912885582069));
#45854=CARTESIAN_POINT('Ctrl Pts',(-0.793331499589108,-0.591564275791708,
-0.40448064329371));
#45855=CARTESIAN_POINT('Ctrl Pts',(-0.890944916136291,-0.460657455465276,
-0.411048401005351));
#45856=CARTESIAN_POINT('Ctrl Pts',(-0.955466981039936,-0.305075374224508,
-0.417616158716993));
#45857=CARTESIAN_POINT('Ctrl Pts',(-0.97914697931892,-0.143507331574391,
-0.424183916428634));
#45858=CARTESIAN_POINT('Ctrl Pts',(-0.986106006327955,-0.096026062388788,
-0.426114034951686));
#45859=CARTESIAN_POINT('Ctrl Pts',(-0.989537741278422,-0.0480278204863994,
-0.428044153474738));
#45860=CARTESIAN_POINT('Ctrl Pts',(-0.98949450850966,-2.34504978581795E-5,
-0.429974271997791));
#45861=CARTESIAN_POINT('Ctrl Pts',(-0.989491623038811,-2.31174877268823E-5,
-0.465975728002209));
#45862=CARTESIAN_POINT('Ctrl Pts',(-0.98953496975876,-0.049075798221059,
-0.464003476366476));
#45863=CARTESIAN_POINT('Ctrl Pts',(-0.985951175030704,-0.0981222013734553,
-0.462031224730742));
#45864=CARTESIAN_POINT('Ctrl Pts',(-0.978686144299608,-0.14661711800828,
-0.460058973095008));
#45865=CARTESIAN_POINT('Ctrl Pts',(-0.954493003452389,-0.308109118792077,
-0.453491215383367));
#45866=CARTESIAN_POINT('Ctrl Pts',(-0.889477018634865,-0.463485443199799,
-0.446923457671725));
#45867=CARTESIAN_POINT('Ctrl Pts',(-0.791448235943943,-0.594081508018418,
-0.440355699960084));
#45868=CARTESIAN_POINT('Ctrl Pts',(-0.693419453253019,-0.724677572837039,
-0.433787942248443));
#45869=CARTESIAN_POINT('Ctrl Pts',(-0.562377872688697,-0.830493378066557,
-0.427220184536801));
#45870=CARTESIAN_POINT('Ctrl Pts',(-0.414064866042057,-0.898817798579287,
-0.42065242682516));
#45871=CARTESIAN_POINT('Ctrl Pts',(-0.265751859395417,-0.967142219092016,
-0.414084669113519));
#45872=CARTESIAN_POINT('Ctrl Pts',(-0.100167426666459,-0.997975254887957,
-0.407516911401877));
#45873=CARTESIAN_POINT('Ctrl Pts',(0.0627975998423243,-0.987613087092117,
-0.400949153690236));
#45874=CARTESIAN_POINT('Ctrl Pts',(0.225762626351105,-0.977250919296277,
-0.394381395978595));
#45875=CARTESIAN_POINT('Ctrl Pts',(0.386108246639711,-0.925693547908657,
-0.387813638266953));
#45876=CARTESIAN_POINT('Ctrl Pts',(0.52457294062125,-0.839134302921211,
-0.381245880555312));
#45877=CARTESIAN_POINT('Ctrl Pts',(0.663037634602796,-0.752575057933762,
-0.374678122843671));
#45878=CARTESIAN_POINT('Ctrl Pts',(0.779621402277273,-0.631013939346482,
-0.368110365132029));
#45879=CARTESIAN_POINT('Ctrl Pts',(0.860319617138808,-0.489053478264194,
-0.361542607420388));
#45880=CARTESIAN_POINT('Ctrl Pts',(0.94101783200034,-0.347093017181912,
-0.354974849708746));
#45881=CARTESIAN_POINT('Ctrl Pts',(0.985830494048933,-0.184733213604624,
-0.348407091997105));
#45882=CARTESIAN_POINT('Ctrl Pts',(0.989374481078401,-0.0214775413191292,
-0.341839334285463));
#45883=CARTESIAN_POINT('Ctrl Pts',(0.992918468107869,0.141778130966367,
-0.335271576573822));
#45884=CARTESIAN_POINT('Ctrl Pts',(0.955193780118211,0.30592967196007,-0.328703818862181));
#45885=CARTESIAN_POINT('Ctrl Pts',(0.880732096848492,0.451258375508424,
-0.32213606115054));
#45886=CARTESIAN_POINT('Ctrl Pts',(0.806270413578773,0.596587079056778,
-0.315568303438898));
#45887=CARTESIAN_POINT('Ctrl Pts',(0.695071735028993,0.723092945159784,
-0.309000545727257));
#45888=CARTESIAN_POINT('Ctrl Pts',(0.560493801988416,0.815579454673507,
-0.302432788015615));
#45889=CARTESIAN_POINT('Ctrl Pts',(0.425915868947842,0.908065964187229,
-0.295865030303974));
#45890=CARTESIAN_POINT('Ctrl Pts',(0.267958681416473,0.966533117111669,
-0.289297272592333));
#45891=CARTESIAN_POINT('Ctrl Pts',(0.105596852931962,0.98395754615998,-0.282729514880691));
#45892=CARTESIAN_POINT('Ctrl Pts',(-0.0567649755525518,1.00138197520829,
-0.27616175716905));
#45893=CARTESIAN_POINT('Ctrl Pts',(-0.223531444990207,0.977763680380474,
-0.269593999457409));
#45894=CARTESIAN_POINT('Ctrl Pts',(-0.374669738952996,0.915939809086429,
-0.263026241745767));
#45895=CARTESIAN_POINT('Ctrl Pts',(-0.525808032915786,0.854115937792385,
-0.256458484034126));
#45896=CARTESIAN_POINT('Ctrl Pts',(-0.661318151403709,0.754086490032113,
-0.249890726322485));
#45897=CARTESIAN_POINT('Ctrl Pts',(-0.76492192342027,0.627867505842223,
-0.243322968610843));
#45898=CARTESIAN_POINT('Ctrl Pts',(-0.868525695436832,0.501648521652333,
-0.236755210899202));
#45899=CARTESIAN_POINT('Ctrl Pts',(-0.940223120982031,0.349240001032824,
-0.23018745318756));
#45900=CARTESIAN_POINT('Ctrl Pts',(-0.971401577532646,0.18895001738729,
-0.223619695475919));
#45901=CARTESIAN_POINT('Ctrl Pts',(-0.983497390554236,0.126764845768462,
-0.221071706318016));
#45902=CARTESIAN_POINT('Ctrl Pts',(-0.989494756047049,0.0633934473055932,
-0.218523717160113));
#45903=CARTESIAN_POINT('Ctrl Pts',(-0.989459186063674,1.54013734824731E-5,
-0.215975728002209));
#45904=CARTESIAN_POINT('Origin',(0.,0.,-2.22262968985462));
#45905=CARTESIAN_POINT('',(-0.846841790252493,1.26228372977161E-5,-0.0976296898546191));
#45906=CARTESIAN_POINT('',(-0.8469,-1.79235740772804E-14,-0.0695250000000001));
#45907=CARTESIAN_POINT('',(-0.8469,-1.79235740772804E-14,-2.22262968985462));
#45908=CARTESIAN_POINT('',(-0.644274518039102,-0.549718620818712,-0.0695250000000005));
#45909=CARTESIAN_POINT('Ctrl Pts',(-0.846841790252493,1.26228372976933E-5,
-0.0976296898546191));
#45910=CARTESIAN_POINT('Ctrl Pts',(-0.846796275356015,-0.0846659001015894,
-0.0936520544135628));
#45911=CARTESIAN_POINT('Ctrl Pts',(-0.817058392758087,-0.284133958169113,
-0.0842838244620231));
#45912=CARTESIAN_POINT('Ctrl Pts',(-0.718653225003286,-0.462367489267768,
-0.0749155945104837));
#45913=CARTESIAN_POINT('Ctrl Pts',(-0.644274518039102,-0.549718620818712,
-0.0695250000000004));
#45914=CARTESIAN_POINT('Origin',(0.,0.,-0.0695250000000001));
#45915=CARTESIAN_POINT('Origin',(0.,0.,-2.22262968985462));
#45916=CARTESIAN_POINT('',(-0.846873903394892,-2.00704647690821E-5,-0.347629689854619));
#45917=CARTESIAN_POINT('',(-0.846843672143023,1.31814993880319E-5,-0.298320310145379));
#45918=CARTESIAN_POINT('',(-0.8469,-1.79235740772804E-14,-2.22262968985462));
#45919=CARTESIAN_POINT('Ctrl Pts',(-0.846873903394892,-2.00704647690883E-5,
-0.347629689854619));
#45920=CARTESIAN_POINT('Ctrl Pts',(-0.846910904816649,-0.041105339602276,
-0.345699571331567));
#45921=CARTESIAN_POINT('Ctrl Pts',(-0.833979505501722,-0.221971415046033,
-0.337201695096874));
#45922=CARTESIAN_POINT('Ctrl Pts',(-0.707306548807687,-0.52741796683899,
-0.322136061150539));
#45923=CARTESIAN_POINT('Ctrl Pts',(-0.37170956586924,-0.800177647492136,
-0.302432788015616));
#45924=CARTESIAN_POINT('Ctrl Pts',(0.053190657773669,-0.880694623556987,
-0.282729514880691));
#45925=CARTESIAN_POINT('Ctrl Pts',(0.46531181093922,-0.749624694225347,
-0.263026241745767));
#45926=CARTESIAN_POINT('Ctrl Pts',(0.765641814643713,-0.438457403875131,
-0.243322968610843));
#45927=CARTESIAN_POINT('Ctrl Pts',(0.88202629773607,-0.0219507226429252,
-0.223619695475919));
#45928=CARTESIAN_POINT('Ctrl Pts',(0.786504041346395,0.399829646175967,
-0.203916422340995));
#45929=CARTESIAN_POINT('Ctrl Pts',(0.502023960458353,0.725550879818389,
-0.184213149206071));
#45930=CARTESIAN_POINT('Ctrl Pts',(0.0969330160579518,0.876958594872486,
-0.164509876071146));
#45931=CARTESIAN_POINT('Ctrl Pts',(-0.331446894786887,0.817676781830008,
-0.144806602936223));
#45932=CARTESIAN_POINT('Ctrl Pts',(-0.680195083172024,0.561948494949336,
-0.125103329801299));
#45933=CARTESIAN_POINT('Ctrl Pts',(-0.828114799287869,0.250092093274441,
-0.109377692107431));
#45934=CARTESIAN_POINT('Ctrl Pts',(-0.846871428249427,0.0551528515873726,
-0.100219812125204));
#45935=CARTESIAN_POINT('Ctrl Pts',(-0.846841790252493,1.26228372976933E-5,
-0.0976296898546191));
#45936=CARTESIAN_POINT('',(-0.729452881030877,0.430276776454125,-0.0695250000000001));
#45937=CARTESIAN_POINT('Origin',(0.,0.,-0.0695250000000001));
#45938=CARTESIAN_POINT('Ctrl Pts',(-0.846843672143023,1.31814993879972E-5,
-0.298320310145379));
#45939=CARTESIAN_POINT('Ctrl Pts',(-0.846795644364765,-0.0855619705691921,
-0.294300541591641));
#45940=CARTESIAN_POINT('Ctrl Pts',(-0.81282103441623,-0.310992633879406,
-0.283713015326262));
#45941=CARTESIAN_POINT('Ctrl Pts',(-0.615791113824046,-0.631865040078709,
-0.266557731349242));
#45942=CARTESIAN_POINT('Ctrl Pts',(-0.241553908007489,-0.848589468760584,
-0.246854458214317));
#45943=CARTESIAN_POINT('Ctrl Pts',(0.190717468786097,-0.861440191483295,
-0.227151185079393));
#45944=CARTESIAN_POINT('Ctrl Pts',(0.577167311767125,-0.667330005151926,
-0.207447911944469));
#45945=CARTESIAN_POINT('Ctrl Pts',(0.824955967175025,-0.312893524930918,
-0.187744638809545));
#45946=CARTESIAN_POINT('Ctrl Pts',(0.874542449448201,0.116715157342132,
-0.168041365674621));
#45947=CARTESIAN_POINT('Ctrl Pts',(0.714032896413046,0.518283961256023,
-0.148338092539697));
#45948=CARTESIAN_POINT('Ctrl Pts',(0.381951553088681,0.795333171794517,
-0.128634819404772));
#45949=CARTESIAN_POINT('Ctrl Pts',(-0.0418431784879791,0.88130717347886,
-0.108931546269849));
#45950=CARTESIAN_POINT('Ctrl Pts',(-0.455688651728263,0.755540682228038,
-0.0892282731349243));
#45951=CARTESIAN_POINT('Ctrl Pts',(-0.658428920058076,0.550684467012711,
-0.0760927577116414));
#45952=CARTESIAN_POINT('Ctrl Pts',(-0.729452881030877,0.430276776454125,
-0.0695250000000001));
#45953=CARTESIAN_POINT('Origin',(0.,0.,-2.22262968985462));
#45954=CARTESIAN_POINT('',(-0.846969994573332,2.57076813978431E-6,-0.59762968985462));
#45955=CARTESIAN_POINT('',(-0.846871433820842,-1.97854529844221E-5,-0.54832031014538));
#45956=CARTESIAN_POINT('',(-0.8469,-1.79235740772804E-14,-2.22262968985462));
#45957=CARTESIAN_POINT('Ctrl Pts',(-0.846969994573332,2.57076813976785E-6,
-0.59762968985462));
#45958=CARTESIAN_POINT('Ctrl Pts',(-0.846945860058509,-0.137257353648154,
-0.591179330537931));
#45959=CARTESIAN_POINT('Ctrl Pts',(-0.778268067817394,-0.41429865733857,
-0.5781612135096));
#45960=CARTESIAN_POINT('Ctrl Pts',(-0.490329529944689,-0.733504750596127,
-0.558575338769629));
#45961=CARTESIAN_POINT('Ctrl Pts',(-0.0828633950269074,-0.878399638460791,
-0.538872065634705));
#45962=CARTESIAN_POINT('Ctrl Pts',(0.344510672939591,-0.812258987832161,
-0.51916879249978));
#45963=CARTESIAN_POINT('Ctrl Pts',(0.689116041785277,-0.550973091934125,
-0.499465519364857));
#45964=CARTESIAN_POINT('Ctrl Pts',(0.868161261709926,-0.157315894794747,
-0.479762246229933));
#45965=CARTESIAN_POINT('Ctrl Pts',(0.838630713437117,0.274136450605954,
-0.460058973095008));
#45966=CARTESIAN_POINT('Ctrl Pts',(0.607619112085,0.639727505843516,-0.440355699960084));
#45967=CARTESIAN_POINT('Ctrl Pts',(0.230627001460258,0.851624009324031,
-0.42065242682516));
#45968=CARTESIAN_POINT('Ctrl Pts',(-0.201773252809055,0.858917820012625,
-0.400949153690236));
#45969=CARTESIAN_POINT('Ctrl Pts',(-0.585697477490385,0.659856599597445,
-0.381245880555312));
#45970=CARTESIAN_POINT('Ctrl Pts',(-0.805083150423093,0.337294247548553,
-0.363472725943439));
#45971=CARTESIAN_POINT('Ctrl Pts',(-0.846784997329527,0.098698558443348,
-0.352267329043209));
#45972=CARTESIAN_POINT('Ctrl Pts',(-0.846873903394892,-2.00704647690883E-5,
-0.347629689854619));
#45973=CARTESIAN_POINT('Ctrl Pts',(-0.846871433820842,-1.97854529844013E-5,
-0.54832031014538));
#45974=CARTESIAN_POINT('Ctrl Pts',(-0.846908532769453,-0.0420022672629993,
-0.546348058509646));
#45975=CARTESIAN_POINT('Ctrl Pts',(-0.833627112812173,-0.223766549843529,
-0.537808049162271));
#45976=CARTESIAN_POINT('Ctrl Pts',(-0.705627497577025,-0.529662242982048,
-0.522700282103254));
#45977=CARTESIAN_POINT('Ctrl Pts',(-0.369165716682379,-0.801354435040497,
-0.502997008968331));
#45978=CARTESIAN_POINT('Ctrl Pts',(0.0559881381817874,-0.88052120096025,
-0.483293735833406));
#45979=CARTESIAN_POINT('Ctrl Pts',(0.467690841465955,-0.748142722918232,
-0.463590462698483));
#45980=CARTESIAN_POINT('Ctrl Pts',(0.767030806126306,-0.436022934136046,
-0.443887189563558));
#45981=CARTESIAN_POINT('Ctrl Pts',(0.882091598392154,-0.0191486227757228,
-0.424183916428634));
#45982=CARTESIAN_POINT('Ctrl Pts',(0.785229856874429,0.402326145625984,
-0.40448064329371));
#45983=CARTESIAN_POINT('Ctrl Pts',(0.499716623159844,0.727142046192322,
-0.384777370158786));
#45984=CARTESIAN_POINT('Ctrl Pts',(0.0941464492269416,0.877262048653223,
-0.365074097023862));
#45985=CARTESIAN_POINT('Ctrl Pts',(-0.3340423978464,0.816619819635224,-0.345370823888938));
#45986=CARTESIAN_POINT('Ctrl Pts',(-0.681977576889138,0.559784653343796,
-0.325667550754014));
#45987=CARTESIAN_POINT('Ctrl Pts',(-0.828510399589799,0.248297168818575,
-0.309984046172828));
#45988=CARTESIAN_POINT('Ctrl Pts',(-0.846874115253527,0.0542562446861801,
-0.300868299303283));
#45989=CARTESIAN_POINT('Ctrl Pts',(-0.846843672143023,1.31814993879972E-5,
-0.298320310145379));
#45990=CARTESIAN_POINT('Origin',(0.,0.,-2.22262968985462));
#45991=CARTESIAN_POINT('',(-0.846860825277875,1.81094851073512E-5,-0.84762968985462));
#45992=CARTESIAN_POINT('',(-0.846970387335345,1.65112873686153E-6,-0.79832031014538));
#45993=CARTESIAN_POINT('',(-0.8469,-1.79235740772804E-14,-2.22262968985462));
#45994=CARTESIAN_POINT('Ctrl Pts',(-0.846860825277874,1.81094851073073E-5,
-0.84762968985462));
#45995=CARTESIAN_POINT('Ctrl Pts',(-0.846786462338563,-0.093706696417362,
-0.843226847455935));
#45996=CARTESIAN_POINT('Ctrl Pts',(-0.808105529948621,-0.327301471617268,
-0.83225624734561));
#45997=CARTESIAN_POINT('Ctrl Pts',(-0.597286702753671,-0.649384987350965,
-0.814717889523642));
#45998=CARTESIAN_POINT('Ctrl Pts',(-0.21694648727339,-0.855211370798415,
-0.795014616388718));
#45999=CARTESIAN_POINT('Ctrl Pts',(0.215515128035896,-0.855573197728189,
-0.775311343253795));
#46000=CARTESIAN_POINT('Ctrl Pts',(0.596199227614297,-0.650383539209966,
-0.75560807011887));
#46001=CARTESIAN_POINT('Ctrl Pts',(0.833646445550691,-0.288939216624994,
-0.735904796983946));
#46002=CARTESIAN_POINT('Ctrl Pts',(0.870810080882589,0.141922761093581,
-0.716201523849022));
#46003=CARTESIAN_POINT('Ctrl Pts',(0.698761569148873,0.538687791363206,
-0.696498250714097));
#46004=CARTESIAN_POINT('Ctrl Pts',(0.358835570259291,0.806033064210061,
-0.676794977579174));
#46005=CARTESIAN_POINT('Ctrl Pts',(-0.0673006847419141,0.879728870116488,
-0.657091704444249));
#46006=CARTESIAN_POINT('Ctrl Pts',(-0.477267948291393,0.742069789586453,
-0.637388431309326));
#46007=CARTESIAN_POINT('Ctrl Pts',(-0.772571573488883,0.426128420690425,
-0.617685158174401));
#46008=CARTESIAN_POINT('Ctrl Pts',(-0.846354016015757,0.144756787875129,
-0.604432244356166));
#46009=CARTESIAN_POINT('Ctrl Pts',(-0.846970433828444,0.00250074087411703,
-0.597747088249572));
#46010=CARTESIAN_POINT('Ctrl Pts',(-0.846969994573332,2.57076813976785E-6,
-0.59762968985462));
#46011=CARTESIAN_POINT('Ctrl Pts',(-0.846970387335345,1.65112873682055E-6,
-0.79832031014538));
#46012=CARTESIAN_POINT('Ctrl Pts',(-0.846954510280718,-0.138154651200368,
-0.791827817716009));
#46013=CARTESIAN_POINT('Ctrl Pts',(-0.777569601086075,-0.416084227657901,
-0.778767567574997));
#46014=CARTESIAN_POINT('Ctrl Pts',(-0.487996886622684,-0.73505870214776,
-0.759139559722345));
#46015=CARTESIAN_POINT('Ctrl Pts',(-0.0800725146138843,-0.878658437255334,
-0.739436286587419));
#46016=CARTESIAN_POINT('Ctrl Pts',(0.347089281341945,-0.811160457452224,
-0.719733013452496));
#46017=CARTESIAN_POINT('Ctrl Pts',(0.690862867437646,-0.548781154334267,
-0.700029740317572));
#46018=CARTESIAN_POINT('Ctrl Pts',(0.868656629691441,-0.154557163048435,
-0.680326467182648));
#46019=CARTESIAN_POINT('Ctrl Pts',(0.837755611590708,0.276799191120675,
-0.660623194047723));
#46020=CARTESIAN_POINT('Ctrl Pts',(0.605583783625261,0.641654531633949,
-0.6409199209128));
#46021=CARTESIAN_POINT('Ctrl Pts',(0.227920434166312,0.852352352402625,
-0.621216647777875));
#46022=CARTESIAN_POINT('Ctrl Pts',(-0.204500806181377,0.858272495905586,
-0.601513374642951));
#46023=CARTESIAN_POINT('Ctrl Pts',(-0.587790721937716,0.657992647495812,
-0.581810101508027));
#46024=CARTESIAN_POINT('Ctrl Pts',(-0.805632939903566,0.335501306150746,
-0.564079080008836));
#46025=CARTESIAN_POINT('Ctrl Pts',(-0.846784990265332,0.0978027980064761,
-0.552915816221287));
#46026=CARTESIAN_POINT('Ctrl Pts',(-0.846871433820842,-1.97854529844013E-5,
-0.54832031014538));
#46027=CARTESIAN_POINT('Origin',(0.,0.,-2.22262968985462));
#46028=CARTESIAN_POINT('',(-0.846851569986366,-1.59002605872431E-5,-1.09762968985462));
#46029=CARTESIAN_POINT('',(-0.846863041881276,1.85264865106838E-5,-1.04832031014538));
#46030=CARTESIAN_POINT('',(-0.8469,-1.79235740772804E-14,-2.22262968985462));
#46031=CARTESIAN_POINT('Ctrl Pts',(-0.846851569986366,-1.59002605872524E-5,
-1.09762968985462));
#46032=CARTESIAN_POINT('Ctrl Pts',(-0.846885954129866,-0.050156087623229,
-1.09527436437394));
#46033=CARTESIAN_POINT('Ctrl Pts',(-0.830285463477599,-0.240088244909022,
-1.08635128118162));
#46034=CARTESIAN_POINT('Ctrl Pts',(-0.690037039814528,-0.549819198252638,
-1.07086044027766));
#46035=CARTESIAN_POINT('Ctrl Pts',(-0.345869372375964,-0.811681368725081,
-1.05115716714273));
#46036=CARTESIAN_POINT('Ctrl Pts',(0.0813934217585064,-0.878537066934349,
-1.03145389400781));
#46037=CARTESIAN_POINT('Ctrl Pts',(0.489101443966296,-0.734324209456049,
-1.01175062087288));
#46038=CARTESIAN_POINT('Ctrl Pts',(0.779302830144596,-0.413689939461657,
-0.99204734773796));
#46039=CARTESIAN_POINT('Ctrl Pts',(0.882276688888196,0.00633335042843485,
-0.972344074603035));
#46040=CARTESIAN_POINT('Ctrl Pts',(0.773283547661882,0.424835052695301,
-0.952640801468111));
#46041=CARTESIAN_POINT('Ctrl Pts',(0.478509011791072,0.74127012129041,-0.932937528333187));
#46042=CARTESIAN_POINT('Ctrl Pts',(0.0687726720265907,0.879615021850747,
-0.913234255198264));
#46043=CARTESIAN_POINT('Ctrl Pts',(-0.357486304177214,0.806632388023741,
-0.893530982063338));
#46044=CARTESIAN_POINT('Ctrl Pts',(-0.697859185484572,0.539856299692775,
-0.873827708928416));
#46045=CARTESIAN_POINT('Ctrl Pts',(-0.831977558135312,0.231975349762819,
-0.858527278192175));
#46046=CARTESIAN_POINT('Ctrl Pts',(-0.846897390171971,0.0461033991976785,
-0.849794605167577));
#46047=CARTESIAN_POINT('Ctrl Pts',(-0.846860825277874,1.81094851073073E-5,
-0.84762968985462));
#46048=CARTESIAN_POINT('Ctrl Pts',(-0.846863041881276,1.85264865106838E-5,
-1.04832031014538));
#46049=CARTESIAN_POINT('Ctrl Pts',(-0.846785938008928,-0.0946024683408287,
-1.04387533463401));
#46050=CARTESIAN_POINT('Ctrl Pts',(-0.80757060413725,-0.329094830876242,
-1.03286260141101));
#46051=CARTESIAN_POINT('Ctrl Pts',(-0.595220747044056,-0.651279140802846,
-1.01528211047636));
#46052=CARTESIAN_POINT('Ctrl Pts',(-0.214228592898141,-0.855896236083242,
-0.995578837341434));
#46053=CARTESIAN_POINT('Ctrl Pts',(0.218231986874677,-0.854884235941514,
-0.975875564206509));
#46054=CARTESIAN_POINT('Ctrl Pts',(0.598262325502182,-0.648486273440926,
-0.956172291071585));
#46055=CARTESIAN_POINT('Ctrl Pts',(0.834560123160567,-0.286289465029356,
-0.936469017936662));
#46056=CARTESIAN_POINT('Ctrl Pts',(0.870354827142315,0.144688395618483,
-0.916765744801736));
#46057=CARTESIAN_POINT('Ctrl Pts',(0.697046758782688,0.540904865042945,
-0.897062471666814));
#46058=CARTESIAN_POINT('Ctrl Pts',(0.356273186507159,0.807168925029088,
-0.877359198531888));
#46059=CARTESIAN_POINT('Ctrl Pts',(-0.0700950291095755,0.879510627480251,
-0.857655925396965));
#46060=CARTESIAN_POINT('Ctrl Pts',(-0.479622911959631,0.740549876294596,
-0.83795265226204));
#46061=CARTESIAN_POINT('Ctrl Pts',(-0.77392137636837,0.423671995955202,
-0.818249379127117));
#46062=CARTESIAN_POINT('Ctrl Pts',(-0.846577873754564,0.142962661529076,
-0.805038598421563));
#46063=CARTESIAN_POINT('Ctrl Pts',(-0.846970571392702,0.00160325070015155,
-0.798395575427651));
#46064=CARTESIAN_POINT('Ctrl Pts',(-0.846970387335345,1.65112873682055E-6,
-0.79832031014538));
#46065=CARTESIAN_POINT('Origin',(0.,0.,-2.22262968985462));
#46066=CARTESIAN_POINT('',(-0.846966250199675,-6.62394975969204E-6,-1.34762968985462));
#46067=CARTESIAN_POINT('',(-0.846849704405232,-1.53444222700805E-5,-1.29832031014538));
#46068=CARTESIAN_POINT('',(-0.8469,-1.79235740772804E-14,-2.22262968985462));
#46069=CARTESIAN_POINT('Ctrl Pts',(-0.846966250199675,-6.62394975969871E-6,
-1.34762968985462));
#46070=CARTESIAN_POINT('Ctrl Pts',(-0.846969009911585,-0.00655669690887438,
-1.34732188129194));
#46071=CARTESIAN_POINT('Ctrl Pts',(-0.845306643333083,-0.152865259786774,
-1.34044631501763));
#46072=CARTESIAN_POINT('Ctrl Pts',(-0.766374416668415,-0.437175617499231,
-1.32700299103167));
#46073=CARTESIAN_POINT('Ctrl Pts',(-0.466565539319551,-0.748845020430254,
-1.30729971789674));
#46074=CARTESIAN_POINT('Ctrl Pts',(-0.0546642776836284,-0.880604385530872,
-1.28759644476182));
#46075=CARTESIAN_POINT('Ctrl Pts',(0.37037007824383,-0.800798521621077,
-1.2678931716269));
#46076=CARTESIAN_POINT('Ctrl Pts',(0.706423012183327,-0.52860078976397,
-1.24818989849197));
#46077=CARTESIAN_POINT('Ctrl Pts',(0.872757797056872,-0.129406702917007,
-1.22848662535705));
#46078=CARTESIAN_POINT('Ctrl Pts',(0.829412495997682,0.300877348044562,
-1.20878335222212));
#46079=CARTESIAN_POINT('Ctrl Pts',(0.586800818836326,0.658875607452487,
-1.1890800790872));
#46080=CARTESIAN_POINT('Ctrl Pts',(0.20321022801312,0.858578983154271,-1.16937680595228));
#46081=CARTESIAN_POINT('Ctrl Pts',(-0.229201625955346,0.852008733372195,
-1.14967353281735));
#46082=CARTESIAN_POINT('Ctrl Pts',(-0.606547782672759,0.640743360806779,
-1.12997025968243));
#46083=CARTESIAN_POINT('Ctrl Pts',(-0.810482644113683,0.319195791254851,
-1.11262231202818));
#46084=CARTESIAN_POINT('Ctrl Pts',(-0.846790074929525,0.0896583902123634,
-1.10184212208558));
#46085=CARTESIAN_POINT('Ctrl Pts',(-0.846851569986366,-1.59002605872524E-5,
-1.09762968985462));
#46086=CARTESIAN_POINT('Ctrl Pts',(-0.846849704405232,-1.53444222701221E-5,
-1.29832031014538));
#46087=CARTESIAN_POINT('Ctrl Pts',(-0.84688337735639,-0.0510527828440758,
-1.29592285155202));
#46088=CARTESIAN_POINT('Ctrl Pts',(-0.829902698745262,-0.241883433963255,
-1.28695763524702));
#46089=CARTESIAN_POINT('Ctrl Pts',(-0.688286911759098,-0.552008499986543,
-1.27142466123037));
#46090=CARTESIAN_POINT('Ctrl Pts',(-0.343289110846343,-0.812776010553405,
-1.25172138809545));
#46091=CARTESIAN_POINT('Ctrl Pts',(0.0841839088554315,-0.878274061125737,
-1.23201811496052));
#46092=CARTESIAN_POINT('Ctrl Pts',(0.49143174202491,-0.732766743163866,
-1.2123148418256));
#46093=CARTESIAN_POINT('Ctrl Pts',(0.78061308498908,-0.411212194007425,
-1.19261156869067));
#46094=CARTESIAN_POINT('Ctrl Pts',(0.882252111754334,0.00913609662776034,
-1.17290829555575));
#46095=CARTESIAN_POINT('Ctrl Pts',(0.771930043206802,0.42728943978447,-1.15320502242083));
#46096=CARTESIAN_POINT('Ctrl Pts',(0.476151759499167,0.742786482700393,
-1.1335017492859));
#46097=CARTESIAN_POINT('Ctrl Pts',(0.0659780018290307,0.879829051709039,
-1.11379847615098));
#46098=CARTESIAN_POINT('Ctrl Pts',(-0.360046972684807,0.805492665650708,
-1.09409520301605));
#46099=CARTESIAN_POINT('Ctrl Pts',(-0.699570651619342,0.537636643421434,
-1.07439192988113));
#46100=CARTESIAN_POINT('Ctrl Pts',(-0.832343654483411,0.230180174733228,
-1.05913363225757));
#46101=CARTESIAN_POINT('Ctrl Pts',(-0.846899864295118,0.0452065737723092,
-1.05044309234566));
#46102=CARTESIAN_POINT('Ctrl Pts',(-0.846863041881276,1.85264865106838E-5,
-1.04832031014538));
#46103=CARTESIAN_POINT('Origin',(0.,0.,-2.22262968985462));
#46104=CARTESIAN_POINT('',(-0.84688555437138,2.10899746275484E-5,-1.59762968985462));
#46105=CARTESIAN_POINT('',(-0.846965023971566,-7.48627396990331E-6,-1.54832031014538));
#46106=CARTESIAN_POINT('',(-0.8469,-1.79235740772804E-14,-2.22262968985462));
#46107=CARTESIAN_POINT('Ctrl Pts',(-0.846885554371379,2.10899746275542E-5,
-1.59762968985462));
#46108=CARTESIAN_POINT('Ctrl Pts',(-0.846786579154185,-0.10274664313416,
-1.59280164049831));
#46109=CARTESIAN_POINT('Ctrl Pts',(-0.802557679176094,-0.345395880262735,
-1.58140583343035));
#46110=CARTESIAN_POINT('Ctrl Pts',(-0.576164155731512,-0.668196828584006,
-1.56344226865076));
#46111=CARTESIAN_POINT('Ctrl Pts',(-0.189421752756959,-0.861726031055052,
-1.54373899551583));
#46112=CARTESIAN_POINT('Ctrl Pts',(0.242829229569888,-0.848225317583151,
-1.52403572238091));
#46113=CARTESIAN_POINT('Ctrl Pts',(0.616740483602872,-0.630938554242118,
-1.50433244924599));
#46114=CARTESIAN_POINT('Ctrl Pts',(0.842479818084434,-0.262068730894017,
-1.48462917611106));
#46115=CARTESIAN_POINT('Ctrl Pts',(0.865813352240911,0.169763085262774,
-1.46492590297614));
#46116=CARTESIAN_POINT('Ctrl Pts',(0.681135203387868,0.560809329104389,
-1.44522262984121));
#46117=CARTESIAN_POINT('Ctrl Pts',(0.332814302334667,0.81712110846086,-1.42551935670629));
#46118=CARTESIAN_POINT('Ctrl Pts',(-0.0954652444970479,0.877119521452837,
-1.40581608357137));
#46119=CARTESIAN_POINT('Ctrl Pts',(-0.500809263564396,0.726389942318086,
-1.38611281043644));
#46120=CARTESIAN_POINT('Ctrl Pts',(-0.781381130347438,0.406226199993855,
-1.36671734586419));
#46121=CARTESIAN_POINT('Ctrl Pts',(-0.846910125522463,0.133203197406965,
-1.35388963900359));
#46122=CARTESIAN_POINT('Ctrl Pts',(-0.846966250199675,-6.62394975969871E-6,
-1.34762968985462));
#46123=CARTESIAN_POINT('Ctrl Pts',(-0.846965023971566,-7.48627396995969E-6,
-1.54832031014538));
#46124=CARTESIAN_POINT('Ctrl Pts',(-0.846968518185878,-0.00745417022599956,
-1.54797036847002));
#46125=CARTESIAN_POINT('Ctrl Pts',(-0.845066969761898,-0.154659544089421,
-1.54105266908302));
#46126=CARTESIAN_POINT('Ctrl Pts',(-0.764981744407948,-0.439607995293088,
-1.52756721198439));
#46127=CARTESIAN_POINT('Ctrl Pts',(-0.464184283631377,-0.75032340121505,
-1.50786393884946));
#46128=CARTESIAN_POINT('Ctrl Pts',(-0.05186653586545,-0.880773591887012,
-1.48816066571454));
#46129=CARTESIAN_POINT('Ctrl Pts',(0.372912148917511,-0.799617899892882,
-1.46845739257961));
#46130=CARTESIAN_POINT('Ctrl Pts',(0.708098679019178,-0.526353985277906,
-1.44875411944469));
#46131=CARTESIAN_POINT('Ctrl Pts',(0.87316448112032,-0.126633510049379,
-1.42905084630976));
#46132=CARTESIAN_POINT('Ctrl Pts',(0.828452491394789,0.303510669391465,
-1.40934757317484));
#46133=CARTESIAN_POINT('Ctrl Pts',(0.584704766718826,0.660736401868303,
-1.38964430003992));
#46134=CARTESIAN_POINT('Ctrl Pts',(0.200481704953546,0.859220194666598,
-1.36994102690499));
#46135=CARTESIAN_POINT('Ctrl Pts',(-0.231907092208531,0.851276310927182,
-1.35023775377007));
#46136=CARTESIAN_POINT('Ctrl Pts',(-0.608580203776492,0.638813268902558,
-1.33053448063514));
#46137=CARTESIAN_POINT('Ctrl Pts',(-0.810999741514778,0.317401987448,-1.31322866609358));
#46138=CARTESIAN_POINT('Ctrl Pts',(-0.846791131431787,0.0887625744285762,
-1.30249060926366));
#46139=CARTESIAN_POINT('Ctrl Pts',(-0.846849704405232,-1.53444222701221E-5,
-1.29832031014538));
#46140=CARTESIAN_POINT('Origin',(9.02152032747242E-17,0.,-0.0695250000000002));
#46141=CARTESIAN_POINT('',(0.924091453827287,-0.353856906938908,-0.0695250000000001));
#46142=CARTESIAN_POINT('Ctrl Pts',(-0.644274518039098,-0.549718620818717,
-0.0695250000000001));
#46143=CARTESIAN_POINT('Ctrl Pts',(-0.629514607897228,-0.570212568079803,
-0.0695250000000002));
#46144=CARTESIAN_POINT('Ctrl Pts',(-0.613856197663174,-0.590011328072283,
-0.0695250000000003));
#46145=CARTESIAN_POINT('Ctrl Pts',(-0.597342646439648,-0.609050847410868,
-0.0695250000000002));
#46146=CARTESIAN_POINT('Ctrl Pts',(-0.573764312529119,-0.636235802263072,
-0.069525));
#46147=CARTESIAN_POINT('Ctrl Pts',(-0.548443954816583,-0.661874145350851,
-0.0695250000000003));
#46148=CARTESIAN_POINT('Ctrl Pts',(-0.521577921430738,-0.685866619007268,
-0.0695250000000004));
#46149=CARTESIAN_POINT('Ctrl Pts',(-0.513406905541179,-0.693163672526888,
-0.0695250000000004));
#46150=CARTESIAN_POINT('Ctrl Pts',(-0.505092690910161,-0.700308333369332,
-0.0695250000000004));
#46151=CARTESIAN_POINT('Ctrl Pts',(-0.496640257082355,-0.707297384869979,
-0.0695250000000004));
#46152=CARTESIAN_POINT('Ctrl Pts',(-0.489314977156243,-0.713354428285312,
-0.0695250000000004));
#46153=CARTESIAN_POINT('Ctrl Pts',(-0.481887585227203,-0.719293024959345,
-0.069525));
#46154=CARTESIAN_POINT('Ctrl Pts',(-0.474370457275395,-0.72510452921095,
-0.0695249999999999));
#46155=CARTESIAN_POINT('Ctrl Pts',(-0.442888567313103,-0.749443231244141,
-0.0695249999999998));
#46156=CARTESIAN_POINT('Ctrl Pts',(-0.409793969953919,-0.771590511960091,
-0.0695250000000001));
#46157=CARTESIAN_POINT('Ctrl Pts',(-0.375343642665579,-0.791414612519383,
-0.0695250000000003));
#46158=CARTESIAN_POINT('Ctrl Pts',(-0.350727952172436,-0.80557946847527,
-0.0695250000000005));
#46159=CARTESIAN_POINT('Ctrl Pts',(-0.325419068593534,-0.818557693233704,
-0.0695250000000005));
#46160=CARTESIAN_POINT('Ctrl Pts',(-0.299499852848171,-0.830289403880256,
-0.0695250000000005));
#46161=CARTESIAN_POINT('Ctrl Pts',(-0.291030362789716,-0.834122915189619,
-0.0695250000000005));
#46162=CARTESIAN_POINT('Ctrl Pts',(-0.282504034872275,-0.837819395972558,
-0.0695249999999998));
#46163=CARTESIAN_POINT('Ctrl Pts',(-0.273927638577144,-0.84137590496099,
-0.0695249999999998));
#46164=CARTESIAN_POINT('Ctrl Pts',(-0.264547191210553,-0.845265842439012,
-0.0695249999999998));
#46165=CARTESIAN_POINT('Ctrl Pts',(-0.255105521084919,-0.848988937674037,
-0.069525));
#46166=CARTESIAN_POINT('Ctrl Pts',(-0.245606840153278,-0.852543254107393,
-0.069525));
#46167=CARTESIAN_POINT('Ctrl Pts',(-0.207900418576629,-0.86665263990711,
-0.069525));
#46168=CARTESIAN_POINT('Ctrl Pts',(-0.169298093448506,-0.878105947076264,
-0.0695249999999999));
#46169=CARTESIAN_POINT('Ctrl Pts',(-0.130091573045686,-0.88693130443109,
-0.0695249999999997));
#46170=CARTESIAN_POINT('Ctrl Pts',(-0.102099247085215,-0.893232355308744,
-0.0695249999999996));
#46171=CARTESIAN_POINT('Ctrl Pts',(-0.073798080309421,-0.898192899460623,
-0.0695249999999996));
#46172=CARTESIAN_POINT('Ctrl Pts',(-0.0452868955746615,-0.90180864777946,
-0.0695249999999996));
#46173=CARTESIAN_POINT('Ctrl Pts',(-0.0239859768418001,-0.904510000312319,
-0.0695249999999995));
#46174=CARTESIAN_POINT('Ctrl Pts',(-0.00256769535849218,-0.906460483102193,
-0.0695249999999999));
#46175=CARTESIAN_POINT('Ctrl Pts',(0.0189277734581549,-0.907653646015335,
-0.0695249999999999));
#46176=CARTESIAN_POINT('Ctrl Pts',(0.026864202214143,-0.908094178507797,
-0.0695249999999999));
#46177=CARTESIAN_POINT('Ctrl Pts',(0.0348136815882982,-0.908431500832323,
-0.0695249999999997));
#46178=CARTESIAN_POINT('Ctrl Pts',(0.042765812934101,-0.908664920818656,
-0.0695249999999997));
#46179=CARTESIAN_POINT('Ctrl Pts',(0.0842470804049054,-0.909882526070012,
-0.0695249999999998));
#46180=CARTESIAN_POINT('Ctrl Pts',(0.125677974715032,-0.908275201452815,
-0.0695250000000009));
#46181=CARTESIAN_POINT('Ctrl Pts',(0.166763121040939,-0.903860943778449,
-0.0695250000000008));
#46182=CARTESIAN_POINT('Ctrl Pts',(0.176627678125244,-0.902801079065587,
-0.0695250000000008));
#46183=CARTESIAN_POINT('Ctrl Pts',(0.186472385882437,-0.901579177917462,
-0.0695250000000002));
#46184=CARTESIAN_POINT('Ctrl Pts',(0.196293280785995,-0.900195063374112,
-0.0695250000000002));
#46185=CARTESIAN_POINT('Ctrl Pts',(0.234668994651919,-0.89478655588117,
-0.0695250000000001));
#46186=CARTESIAN_POINT('Ctrl Pts',(0.272681208109324,-0.886904450937793,
-0.0695250000000005));
#46187=CARTESIAN_POINT('Ctrl Pts',(0.310125123955116,-0.876660725787972,
-0.0695250000000006));
#46188=CARTESIAN_POINT('Ctrl Pts',(0.329782155791864,-0.871283050220432,
-0.0695250000000006));
#46189=CARTESIAN_POINT('Ctrl Pts',(0.349282561029609,-0.865253829412173,
-0.0695250000000006));
#46190=CARTESIAN_POINT('Ctrl Pts',(0.36859600834363,-0.858584870376398,
-0.0695250000000006));
#46191=CARTESIAN_POINT('Ctrl Pts',(0.376732359496032,-0.855775377505767,
-0.0695250000000006));
#46192=CARTESIAN_POINT('Ctrl Pts',(0.384837496765632,-0.852851562967871,
-0.0695250000000003));
#46193=CARTESIAN_POINT('Ctrl Pts',(0.392902786498845,-0.849816543883558,
-0.0695250000000003));
#46194=CARTESIAN_POINT('Ctrl Pts',(0.433999942212729,-0.834351426568682,
-0.0695250000000003));
#46195=CARTESIAN_POINT('Ctrl Pts',(0.473890548978183,-0.81607027944879,
-0.0695250000000002));
#46196=CARTESIAN_POINT('Ctrl Pts',(0.51229280876073,-0.795158465405007,
-0.0695250000000002));
#46197=CARTESIAN_POINT('Ctrl Pts',(0.550695068543278,-0.774246651361224,
-0.0695250000000001));
#46198=CARTESIAN_POINT('Ctrl Pts',(0.5876103412066,-0.750703718346156,-0.0695250000000004));
#46199=CARTESIAN_POINT('Ctrl Pts',(0.622745109445882,-0.724656753629564,
-0.0695250000000004));
#46200=CARTESIAN_POINT('Ctrl Pts',(0.638877111365698,-0.712697383869337,
-0.0695250000000005));
#46201=CARTESIAN_POINT('Ctrl Pts',(0.654633463274635,-0.700209354343849,
-0.0695250000000005));
#46202=CARTESIAN_POINT('Ctrl Pts',(0.669996947566329,-0.687216016520921,
-0.0695250000000005));
#46203=CARTESIAN_POINT('Ctrl Pts',(0.678922789820835,-0.679667176585591,
-0.0695250000000005));
#46204=CARTESIAN_POINT('Ctrl Pts',(0.68771599710606,-0.671947736058525,
-0.0695250000000001));
#46205=CARTESIAN_POINT('Ctrl Pts',(0.696372929515829,-0.66406195754111,
-0.0695250000000001));
#46206=CARTESIAN_POINT('Ctrl Pts',(0.702557911261651,-0.658427929934892,
-0.0695250000000001));
#46207=CARTESIAN_POINT('Ctrl Pts',(0.708673069158198,-0.652709060668137,
-0.0695250000000001));
#46208=CARTESIAN_POINT('Ctrl Pts',(0.714707061246942,-0.646916923963097,
-0.0695250000000001));
#46209=CARTESIAN_POINT('Ctrl Pts',(0.745695686752405,-0.617170389233001,
-0.0695250000000001));
#46210=CARTESIAN_POINT('Ctrl Pts',(0.77461545607891,-0.585432521388643,
-0.069525));
#46211=CARTESIAN_POINT('Ctrl Pts',(0.801330866406532,-0.551969355975223,
-0.069525));
#46212=CARTESIAN_POINT('Ctrl Pts',(0.828287682902432,-0.518203810233675,
-0.069525));
#46213=CARTESIAN_POINT('Ctrl Pts',(0.853000960044775,-0.48268086089206,
-0.0695249999999999));
#46214=CARTESIAN_POINT('Ctrl Pts',(0.875301042068569,-0.445631041576752,
-0.0695249999999999));
#46215=CARTESIAN_POINT('Ctrl Pts',(0.893145601953607,-0.41598371925765,
-0.0695249999999999));
#46216=CARTESIAN_POINT('Ctrl Pts',(0.909444522886281,-0.385357711644212,
-0.069525));
#46217=CARTESIAN_POINT('Ctrl Pts',(0.924091453827287,-0.353856906938908,
-0.0695250000000001));
#46218=CARTESIAN_POINT('',(-0.989525,-1.21181862392629E-16,-0.0695250000000003));
#46219=CARTESIAN_POINT('Origin',(0.,0.,-0.0695250000000001));
#46220=CARTESIAN_POINT('',(0.849186560444991,0.508032827447782,-0.0695250000000002));
#46221=CARTESIAN_POINT('Origin',(0.,0.,-0.0695250000000001));
#46222=CARTESIAN_POINT('Ctrl Pts',(0.849186560444991,0.508032827447782,
-0.0695250000000002));
#46223=CARTESIAN_POINT('Ctrl Pts',(0.832465613029651,0.532075780979081,
-0.0695250000000002));
#46224=CARTESIAN_POINT('Ctrl Pts',(0.814699598175689,0.555333492117173,
-0.0695249999999997));
#46225=CARTESIAN_POINT('Ctrl Pts',(0.795920427116913,0.577725594506868,
-0.0695249999999998));
#46226=CARTESIAN_POINT('Ctrl Pts',(0.770244398979351,0.60834144273667,-0.0695249999999999));
#46227=CARTESIAN_POINT('Ctrl Pts',(0.742674876881569,0.637340509727314,
-0.0695250000000005));
#46228=CARTESIAN_POINT('Ctrl Pts',(0.713391010537452,0.66457844663845,-0.0695250000000007));
#46229=CARTESIAN_POINT('Ctrl Pts',(0.703372076901965,0.67389740333199,-0.0695250000000007));
#46230=CARTESIAN_POINT('Ctrl Pts',(0.693152303997172,0.683009942300558,
-0.0695250000000002));
#46231=CARTESIAN_POINT('Ctrl Pts',(0.68273841510423,0.691909392025286,-0.0695250000000002));
#46232=CARTESIAN_POINT('Ctrl Pts',(0.675105784312335,0.698432047941648,
-0.0695250000000002));
#46233=CARTESIAN_POINT('Ctrl Pts',(0.667370342782135,0.704838817597991,
-0.0695250000000004));
#46234=CARTESIAN_POINT('Ctrl Pts',(0.659543833079429,0.711120248251889,
-0.0695250000000004));
#46235=CARTESIAN_POINT('Ctrl Pts',(0.626058981692227,0.737994650754968,
-0.0695250000000004));
#46236=CARTESIAN_POINT('Ctrl Pts',(0.590864886279207,0.762616605548979,
-0.069525));
#46237=CARTESIAN_POINT('Ctrl Pts',(0.554186287487196,0.784804033106952,
-0.069525));
#46238=CARTESIAN_POINT('Ctrl Pts',(0.529103291209082,0.799977108992796,
-0.069525));
#46239=CARTESIAN_POINT('Ctrl Pts',(0.503325419420093,0.814010769328655,
-0.0695250000000002));
#46240=CARTESIAN_POINT('Ctrl Pts',(0.47692006115639,0.826833197390815,-0.0695250000000003));
#46241=CARTESIAN_POINT('Ctrl Pts',(0.46840181479615,0.830969653335822,-0.0695250000000004));
#46242=CARTESIAN_POINT('Ctrl Pts',(0.459816463861541,0.834980640477273,
-0.0695249999999996));
#46243=CARTESIAN_POINT('Ctrl Pts',(0.451182152464372,0.838856712876695,
-0.0695249999999997));
#46244=CARTESIAN_POINT('Ctrl Pts',(0.437905879500253,0.844816631720981,
-0.0695249999999997));
#46245=CARTESIAN_POINT('Ctrl Pts',(0.424506188175036,0.8504615084049,-0.069525));
#46246=CARTESIAN_POINT('Ctrl Pts',(0.410992010006838,0.85578480548222,-0.069525));
#46247=CARTESIAN_POINT('Ctrl Pts',(0.371777648040439,0.871231523428853,
-0.0695250000000001));
#46248=CARTESIAN_POINT('Ctrl Pts',(0.331600099063284,0.883974369710503,
-0.0695249999999996));
#46249=CARTESIAN_POINT('Ctrl Pts',(0.290745866776486,0.893985042687368,
-0.0695249999999996));
#46250=CARTESIAN_POINT('Ctrl Pts',(0.25024980796209,0.903907951011698,-0.0695249999999996));
#46251=CARTESIAN_POINT('Ctrl Pts',(0.209087691304592,0.911146366027076,
-0.0695250000000002));
#46252=CARTESIAN_POINT('Ctrl Pts',(0.167537654230177,0.915622168647208,
-0.0695250000000004));
#46253=CARTESIAN_POINT('Ctrl Pts',(0.149988630342492,0.917512563280469,
-0.0695250000000005));
#46254=CARTESIAN_POINT('Ctrl Pts',(0.132370498081357,0.918909523988645,
-0.0695250000000004));
#46255=CARTESIAN_POINT('Ctrl Pts',(0.114704940581103,0.919804424450112,
-0.0695250000000005));
#46256=CARTESIAN_POINT('Ctrl Pts',(0.106506859464303,0.920219722216654,
-0.0695250000000005));
#46257=CARTESIAN_POINT('Ctrl Pts',(0.0983079054751423,0.920526381597904,
-0.069525));
#46258=CARTESIAN_POINT('Ctrl Pts',(0.0901122544371284,0.920724168836828,
-0.069525));
#46259=CARTESIAN_POINT('Ctrl Pts',(0.0489897278813967,0.921716586760351,
-0.0695250000000002));
#46260=CARTESIAN_POINT('Ctrl Pts',(0.00793295039935812,0.919973010373648,
-0.0695249999999997));
#46261=CARTESIAN_POINT('Ctrl Pts',(-0.0327910898782061,0.915446284625334,
-0.0695249999999998));
#46262=CARTESIAN_POINT('Ctrl Pts',(-0.0363378459041664,0.915052041035644,
-0.0695249999999998));
#46263=CARTESIAN_POINT('Ctrl Pts',(-0.0398820734162914,0.914636654549671,
-0.0695250000000006));
#46264=CARTESIAN_POINT('Ctrl Pts',(-0.0434235925645807,0.914200075428631,
-0.0695250000000006));
#46265=CARTESIAN_POINT('Ctrl Pts',(-0.0802746321872905,0.909657280708554,
-0.0695250000000005));
#46266=CARTESIAN_POINT('Ctrl Pts',(-0.116833648576168,0.902822475100424,
-0.0695250000000003));
#46267=CARTESIAN_POINT('Ctrl Pts',(-0.152895642013777,0.89375708945521,
-0.0695250000000002));
#46268=CARTESIAN_POINT('Ctrl Pts',(-0.171831220409218,0.888996999837124,
-0.0695250000000002));
#46269=CARTESIAN_POINT('Ctrl Pts',(-0.190629523232773,0.883621386847789,
-0.069525));
#46270=CARTESIAN_POINT('Ctrl Pts',(-0.209258732975253,0.877635930874417,
-0.069525));
#46271=CARTESIAN_POINT('Ctrl Pts',(-0.217624297379082,0.874948124031094,
-0.069525));
#46272=CARTESIAN_POINT('Ctrl Pts',(-0.225955740196051,0.872137313528728,
-0.0695250000000003));
#46273=CARTESIAN_POINT('Ctrl Pts',(-0.234250054208824,0.869203882116388,
-0.0695250000000003));
#46274=CARTESIAN_POINT('Ctrl Pts',(-0.241741121075245,0.866554533318638,
-0.0695250000000003));
#46275=CARTESIAN_POINT('Ctrl Pts',(-0.249193176417347,0.863808233930807,
-0.069525));
#46276=CARTESIAN_POINT('Ctrl Pts',(-0.256602800192705,0.860966475101326,
-0.069525));
#46277=CARTESIAN_POINT('Ctrl Pts',(-0.294124992514654,0.846575863031793,
-0.069525));
#46278=CARTESIAN_POINT('Ctrl Pts',(-0.330574092810289,0.829736301930517,
-0.0695250000000004));
#46279=CARTESIAN_POINT('Ctrl Pts',(-0.365695559063158,0.810541946680565,
-0.0695250000000003));
#46280=CARTESIAN_POINT('Ctrl Pts',(-0.396561761353498,0.793673150608326,
-0.0695250000000002));
#46281=CARTESIAN_POINT('Ctrl Pts',(-0.426402744048706,0.774984657826367,
-0.0695250000000004));
#46282=CARTESIAN_POINT('Ctrl Pts',(-0.455025122704759,0.754514235939637,
-0.0695250000000004));
#46283=CARTESIAN_POINT('Ctrl Pts',(-0.469941989788981,0.743845850683762,
-0.0695250000000004));
#46284=CARTESIAN_POINT('Ctrl Pts',(-0.484527482772804,0.732693076977225,
-0.0695250000000004));
#46285=CARTESIAN_POINT('Ctrl Pts',(-0.498760924054214,0.721074151458354,
-0.0695250000000004));
#46286=CARTESIAN_POINT('Ctrl Pts',(-0.50875747684214,0.712913847847161,
-0.0695250000000004));
#46287=CARTESIAN_POINT('Ctrl Pts',(-0.518580335702014,0.704523581635438,
-0.0695250000000002));
#46288=CARTESIAN_POINT('Ctrl Pts',(-0.528221721630384,0.695909387857388,
-0.0695250000000001));
#46289=CARTESIAN_POINT('Ctrl Pts',(-0.534327024836865,0.690454542953854,
-0.0695250000000001));
#46290=CARTESIAN_POINT('Ctrl Pts',(-0.540353017486882,0.684915689319018,
-0.0695250000000007));
#46291=CARTESIAN_POINT('Ctrl Pts',(-0.546295490452486,0.679297484790217,
-0.0695250000000007));
#46292=CARTESIAN_POINT('Ctrl Pts',(-0.574958072746145,0.652198960222842,
-0.0695250000000006));
#46293=CARTESIAN_POINT('Ctrl Pts',(-0.601702485869931,0.623237707774714,
-0.0695250000000003));
#46294=CARTESIAN_POINT('Ctrl Pts',(-0.626357124444992,0.59262560076324,
-0.0695250000000003));
#46295=CARTESIAN_POINT('Ctrl Pts',(-0.650560797781831,0.562573428795588,
-0.0695250000000002));
#46296=CARTESIAN_POINT('Ctrl Pts',(-0.672750955666676,0.530929222698942,
-0.0695250000000002));
#46297=CARTESIAN_POINT('Ctrl Pts',(-0.692721855863329,0.497870363939758,
-0.0695250000000001));
#46298=CARTESIAN_POINT('Ctrl Pts',(-0.705966728863737,0.475945444106792,
-0.069525));
#46299=CARTESIAN_POINT('Ctrl Pts',(-0.718234573055067,0.453397852226439,
-0.0695250000000001));
#46300=CARTESIAN_POINT('Ctrl Pts',(-0.729452881030877,0.430276776454125,
-0.0695250000000001));
#46301=CARTESIAN_POINT('Ctrl Pts',(-0.370207279419763,0.761699534110805,
-1.84281958214317));
#46302=CARTESIAN_POINT('Ctrl Pts',(-0.495937788115843,0.700590990019629,
-1.83625182443153));
#46303=CARTESIAN_POINT('Ctrl Pts',(-0.716438090811261,0.514985758881006,
-1.82311630900825));
#46304=CARTESIAN_POINT('Ctrl Pts',(-0.875085689900816,0.112597606289335,
-1.80341303587332));
#46305=CARTESIAN_POINT('Ctrl Pts',(-0.823479197849261,-0.316739409883142,
-1.7837097627384));
#46306=CARTESIAN_POINT('Ctrl Pts',(-0.574039462429418,-0.670029803239366,
-1.76400648960348));
#46307=CARTESIAN_POINT('Ctrl Pts',(-0.186682838485098,-0.862320382256737,
-1.74430321646855));
#46308=CARTESIAN_POINT('Ctrl Pts',(0.2455223736064,-0.847451160704884,-1.72459994333363));
#46309=CARTESIAN_POINT('Ctrl Pts',(0.618741824242655,-0.628975354430863,
-1.7048966701987));
#46310=CARTESIAN_POINT('Ctrl Pts',(0.843308030144031,-0.259391446847321,
-1.68519339706378));
#46311=CARTESIAN_POINT('Ctrl Pts',(0.865269712120719,0.172512904594376,
-1.66549012392885));
#46312=CARTESIAN_POINT('Ctrl Pts',(0.679350192014294,0.562970195790566,
-1.64578685079393));
#46313=CARTESIAN_POINT('Ctrl Pts',(0.330216833785133,0.818174300873478,
-1.626083577659));
#46314=CARTESIAN_POINT('Ctrl Pts',(-0.0982511612190419,0.876811794340843,
-1.60638030452408));
#46315=CARTESIAN_POINT('Ctrl Pts',(-0.503114295254248,0.724795336222326,
-1.58667703138916));
#46316=CARTESIAN_POINT('Ctrl Pts',(-0.78710421375316,0.398646723393102,
-1.56697375825423));
#46317=CARTESIAN_POINT('Ctrl Pts',(-0.88199231792273,-0.023276748797502,
-1.54727048511931));
#46318=CARTESIAN_POINT('Ctrl Pts',(-0.764981744407948,-0.439607995293088,
-1.52756721198439));
#46319=CARTESIAN_POINT('Ctrl Pts',(-0.464184283631377,-0.75032340121505,
-1.50786393884946));
#46320=CARTESIAN_POINT('Ctrl Pts',(-0.05186653586545,-0.880773591887012,
-1.48816066571454));
#46321=CARTESIAN_POINT('Ctrl Pts',(0.372912148917511,-0.799617899892882,
-1.46845739257961));
#46322=CARTESIAN_POINT('Ctrl Pts',(0.708098679019178,-0.526353985277906,
-1.44875411944469));
#46323=CARTESIAN_POINT('Ctrl Pts',(0.87316448112032,-0.126633510049379,
-1.42905084630976));
#46324=CARTESIAN_POINT('Ctrl Pts',(0.828452491394789,0.303510669391465,
-1.40934757317484));
#46325=CARTESIAN_POINT('Ctrl Pts',(0.584704766718826,0.660736401868303,
-1.38964430003992));
#46326=CARTESIAN_POINT('Ctrl Pts',(0.200481704953546,0.859220194666598,
-1.36994102690499));
#46327=CARTESIAN_POINT('Ctrl Pts',(-0.231907092208531,0.851276310927182,
-1.35023775377007));
#46328=CARTESIAN_POINT('Ctrl Pts',(-0.608580203776492,0.638813268902558,
-1.33053448063514));
#46329=CARTESIAN_POINT('Ctrl Pts',(-0.839041903820945,0.272875320594155,
-1.31083120750022));
#46330=CARTESIAN_POINT('Ctrl Pts',(-0.867923762256349,-0.158620931366679,
-1.29112793436529));
#46331=CARTESIAN_POINT('Ctrl Pts',(-0.688286911759098,-0.552008499986543,
-1.27142466123037));
#46332=CARTESIAN_POINT('Ctrl Pts',(-0.343289110846343,-0.812776010553405,
-1.25172138809545));
#46333=CARTESIAN_POINT('Ctrl Pts',(0.0841839088554315,-0.878274061125737,
-1.23201811496052));
#46334=CARTESIAN_POINT('Ctrl Pts',(0.49143174202491,-0.732766743163866,
-1.2123148418256));
#46335=CARTESIAN_POINT('Ctrl Pts',(0.78061308498908,-0.411212194007425,
-1.19261156869067));
#46336=CARTESIAN_POINT('Ctrl Pts',(0.882252111754334,0.00913609662776034,
-1.17290829555575));
#46337=CARTESIAN_POINT('Ctrl Pts',(0.771930043206802,0.42728943978447,-1.15320502242083));
#46338=CARTESIAN_POINT('Ctrl Pts',(0.476151759499167,0.742786482700393,
-1.1335017492859));
#46339=CARTESIAN_POINT('Ctrl Pts',(0.0659780018290307,0.879829051709039,
-1.11379847615098));
#46340=CARTESIAN_POINT('Ctrl Pts',(-0.360046972684807,0.805492665650708,
-1.09409520301605));
#46341=CARTESIAN_POINT('Ctrl Pts',(-0.699570651619342,0.537636643421434,
-1.07439192988113));
#46342=CARTESIAN_POINT('Ctrl Pts',(-0.871022461311121,0.140613402092739,
-1.05468865674621));
#46343=CARTESIAN_POINT('Ctrl Pts',(-0.833211099533203,-0.290192213147162,
-1.03498538361128));
#46344=CARTESIAN_POINT('Ctrl Pts',(-0.595220747044056,-0.651279140802846,
-1.01528211047636));
#46345=CARTESIAN_POINT('Ctrl Pts',(-0.214228592898141,-0.855896236083242,
-0.995578837341434));
#46346=CARTESIAN_POINT('Ctrl Pts',(0.218231986874677,-0.854884235941514,
-0.975875564206509));
#46347=CARTESIAN_POINT('Ctrl Pts',(0.598262325502182,-0.648486273440926,
-0.956172291071585));
#46348=CARTESIAN_POINT('Ctrl Pts',(0.834560123160567,-0.286289465029356,
-0.936469017936662));
#46349=CARTESIAN_POINT('Ctrl Pts',(0.870354827142315,0.144688395618483,
-0.916765744801736));
#46350=CARTESIAN_POINT('Ctrl Pts',(0.697046758782688,0.540904865042945,
-0.897062471666814));
#46351=CARTESIAN_POINT('Ctrl Pts',(0.356273186507159,0.807168925029088,
-0.877359198531888));
#46352=CARTESIAN_POINT('Ctrl Pts',(-0.0700950291095755,0.879510627480251,
-0.857655925396965));
#46353=CARTESIAN_POINT('Ctrl Pts',(-0.479622911959631,0.740549876294596,
-0.83795265226204));
#46354=CARTESIAN_POINT('Ctrl Pts',(-0.77392137636837,0.423671995955202,
-0.818249379127117));
#46355=CARTESIAN_POINT('Ctrl Pts',(-0.88228520776747,0.00500690635942724,
-0.798546105992192));
#46356=CARTESIAN_POINT('Ctrl Pts',(-0.778679992535662,-0.41486109263371,
-0.778842832857268));
#46357=CARTESIAN_POINT('Ctrl Pts',(-0.487996886622684,-0.73505870214776,
-0.759139559722345));
#46358=CARTESIAN_POINT('Ctrl Pts',(-0.0800725146138843,-0.878658437255334,
-0.739436286587419));
#46359=CARTESIAN_POINT('Ctrl Pts',(0.347089281341945,-0.811160457452224,
-0.719733013452496));
#46360=CARTESIAN_POINT('Ctrl Pts',(0.690862867437646,-0.548781154334267,
-0.700029740317572));
#46361=CARTESIAN_POINT('Ctrl Pts',(0.868656629691441,-0.154557163048435,
-0.680326467182648));
#46362=CARTESIAN_POINT('Ctrl Pts',(0.837755611590708,0.276799191120675,
-0.660623194047723));
#46363=CARTESIAN_POINT('Ctrl Pts',(0.605583783625261,0.641654531633949,
-0.6409199209128));
#46364=CARTESIAN_POINT('Ctrl Pts',(0.227920434166312,0.852352352402625,
-0.621216647777875));
#46365=CARTESIAN_POINT('Ctrl Pts',(-0.204500806181377,0.858272495905586,
-0.601513374642951));
#46366=CARTESIAN_POINT('Ctrl Pts',(-0.587790721937716,0.657992647495812,
-0.581810101508027));
#46367=CARTESIAN_POINT('Ctrl Pts',(-0.829863899791275,0.299630046533427,
-0.562106828373103));
#46368=CARTESIAN_POINT('Ctrl Pts',(-0.872562251752902,-0.130718681755497,
-0.542403555238179));
#46369=CARTESIAN_POINT('Ctrl Pts',(-0.705627497577025,-0.529662242982048,
-0.522700282103254));
#46370=CARTESIAN_POINT('Ctrl Pts',(-0.369165716682379,-0.801354435040497,
-0.502997008968331));
#46371=CARTESIAN_POINT('Ctrl Pts',(0.0559881381817874,-0.88052120096025,
-0.483293735833406));
#46372=CARTESIAN_POINT('Ctrl Pts',(0.467690841465955,-0.748142722918232,
-0.463590462698483));
#46373=CARTESIAN_POINT('Ctrl Pts',(0.767030806126306,-0.436022934136046,
-0.443887189563558));
#46374=CARTESIAN_POINT('Ctrl Pts',(0.882091598392154,-0.0191486227757228,
-0.424183916428634));
#46375=CARTESIAN_POINT('Ctrl Pts',(0.785229856874429,0.402326145625984,
-0.40448064329371));
#46376=CARTESIAN_POINT('Ctrl Pts',(0.499716623159844,0.727142046192322,
-0.384777370158786));
#46377=CARTESIAN_POINT('Ctrl Pts',(0.0941464492269416,0.877262048653223,
-0.365074097023862));
#46378=CARTESIAN_POINT('Ctrl Pts',(-0.3340423978464,0.816619819635224,-0.345370823888938));
#46379=CARTESIAN_POINT('Ctrl Pts',(-0.681977576889138,0.559784653343796,
-0.325667550754014));
#46380=CARTESIAN_POINT('Ctrl Pts',(-0.866067568635368,0.168461211957287,
-0.30596427761909));
#46381=CARTESIAN_POINT('Ctrl Pts',(-0.842084910323148,-0.263335048428687,
-0.286261004484165));
#46382=CARTESIAN_POINT('Ctrl Pts',(-0.615791113824046,-0.631865040078709,
-0.266557731349242));
#46383=CARTESIAN_POINT('Ctrl Pts',(-0.241553908007489,-0.848589468760584,
-0.246854458214317));
#46384=CARTESIAN_POINT('Ctrl Pts',(0.190717468786097,-0.861440191483295,
-0.227151185079393));
#46385=CARTESIAN_POINT('Ctrl Pts',(0.577167311767125,-0.667330005151926,
-0.207447911944469));
#46386=CARTESIAN_POINT('Ctrl Pts',(0.824955967175025,-0.312893524930918,
-0.187744638809545));
#46387=CARTESIAN_POINT('Ctrl Pts',(0.874542449448201,0.116715157342132,
-0.168041365674621));
#46388=CARTESIAN_POINT('Ctrl Pts',(0.714032896413046,0.518283961256023,
-0.148338092539697));
#46389=CARTESIAN_POINT('Ctrl Pts',(0.381951553088681,0.795333171794517,
-0.128634819404772));
#46390=CARTESIAN_POINT('Ctrl Pts',(-0.0418431784879791,0.88130717347886,
-0.108931546269849));
#46391=CARTESIAN_POINT('Ctrl Pts',(-0.455688651728263,0.755540682228038,
-0.0892282731349243));
#46392=CARTESIAN_POINT('Ctrl Pts',(-0.658428920058076,0.550684467012711,
-0.0760927577116414));
#46393=CARTESIAN_POINT('Ctrl Pts',(-0.729452881030877,0.430276776454125,
-0.0695250000000001));
#46394=CARTESIAN_POINT('Ctrl Pts',(-0.390989273841475,0.804458378544447,
-1.81537138809545));
#46395=CARTESIAN_POINT('Ctrl Pts',(-0.523777803477758,0.739919438853238,
-1.80880363038381));
#46396=CARTESIAN_POINT('Ctrl Pts',(-0.756656134146546,0.543895053115038,
-1.79566811496052));
#46397=CARTESIAN_POINT('Ctrl Pts',(-0.924209591393358,0.118918397251283,
-1.7759648418256));
#46398=CARTESIAN_POINT('Ctrl Pts',(-0.869706111925403,-0.33451992640795,
-1.75626156869068));
#46399=CARTESIAN_POINT('Ctrl Pts',(-0.606263801520612,-0.70764266610669,
-1.73655829555575));
#46400=CARTESIAN_POINT('Ctrl Pts',(-0.19716248576299,-0.910727689108931,
-1.71685502242083));
#46401=CARTESIAN_POINT('Ctrl Pts',(0.259305043160306,-0.895023767386323,
-1.6971517492859));
#46402=CARTESIAN_POINT('Ctrl Pts',(0.653475579775621,-0.664283580481048,
-1.67744847615098));
#46403=CARTESIAN_POINT('Ctrl Pts',(0.890648057616496,-0.273952672142162,
-1.65774520301605));
#46404=CARTESIAN_POINT('Ctrl Pts',(0.913842582861546,0.18219710698654,-1.63804192988113));
#46405=CARTESIAN_POINT('Ctrl Pts',(0.717486265197291,0.594573149376045,
-1.61833865674621));
#46406=CARTESIAN_POINT('Ctrl Pts',(0.348753920382767,0.864103418700094,
-1.59863538361128));
#46407=CARTESIAN_POINT('Ctrl Pts',(-0.103766598645288,0.926032592612129,
-1.57893211047636));
#46408=CARTESIAN_POINT('Ctrl Pts',(-0.531357171768844,0.765482522757027,
-1.55922883734143));
#46409=CARTESIAN_POINT('Ctrl Pts',(-0.831289177930963,0.421025197405753,
-1.53952556420651));
#46410=CARTESIAN_POINT('Ctrl Pts',(-0.931503930605742,-0.0245834147939755,
-1.51982229107159));
#46411=CARTESIAN_POINT('Ctrl Pts',(-0.807924839340912,-0.464285875534232,
-1.50011901793666));
#46412=CARTESIAN_POINT('Ctrl Pts',(-0.490241780956103,-0.792443633866798,
-1.48041574480174));
#46413=CARTESIAN_POINT('Ctrl Pts',(-0.0547781211284922,-0.930216790038264,
-1.46071247166681));
#46414=CARTESIAN_POINT('Ctrl Pts',(0.393845984175257,-0.844505333660041,
-1.44100919853189));
#46415=CARTESIAN_POINT('Ctrl Pts',(0.747848580264941,-0.555901447453789,
-1.42130592539697));
#46416=CARTESIAN_POINT('Ctrl Pts',(0.922180533436526,-0.133742221967667,
-1.40160265226204));
#46417=CARTESIAN_POINT('Ctrl Pts',(0.874958586795736,0.32054857596129,-1.38189937912712));
#46418=CARTESIAN_POINT('Ctrl Pts',(0.617527814443183,0.697827569387674,
-1.36219610599219));
#46419=CARTESIAN_POINT('Ctrl Pts',(0.211735966837673,0.90745346906512,-1.34249283285727));
#46420=CARTESIAN_POINT('Ctrl Pts',(-0.244925452906858,0.89906364664017,
-1.32278955972234));
#46421=CARTESIAN_POINT('Ctrl Pts',(-0.642743525523892,0.674673757144865,
-1.30308628658742));
#46422=CARTESIAN_POINT('Ctrl Pts',(-0.886142447581508,0.288193478030981,
-1.28338301345249));
#46423=CARTESIAN_POINT('Ctrl Pts',(-0.916645621032203,-0.167525292501866,
-1.26367974031757));
#46424=CARTESIAN_POINT('Ctrl Pts',(-0.726924657573103,-0.582996106673904,
-1.24397646718265));
#46425=CARTESIAN_POINT('Ctrl Pts',(-0.362560024151519,-0.858402089391984,
-1.22427319404772));
#46426=CARTESIAN_POINT('Ctrl Pts',(0.0889096655368591,-0.927576945357665,
-1.2045699209128));
#46427=CARTESIAN_POINT('Ctrl Pts',(0.519018805513831,-0.773901413429442,
-1.18486664777787));
#46428=CARTESIAN_POINT('Ctrl Pts',(0.824433662486056,-0.434296044588096,
-1.16516337464295));
#46429=CARTESIAN_POINT('Ctrl Pts',(0.931778308250955,0.00964896150024885,
-1.14546010150803));
#46430=CARTESIAN_POINT('Ctrl Pts',(0.815263188565314,0.451275804309702,
-1.1257568283731));
#46431=CARTESIAN_POINT('Ctrl Pts',(0.502881064296495,0.78448362210888,-1.10605355523818));
#46432=CARTESIAN_POINT('Ctrl Pts',(0.0696817498161479,0.929219227054417,
-1.08635028210326));
#46433=CARTESIAN_POINT('Ctrl Pts',(-0.380258607068705,0.850709885880736,
-1.06664700896833));
#46434=CARTESIAN_POINT('Ctrl Pts',(-0.738841822630168,0.567817470070777,
-1.04694373583341));
#46435=CARTESIAN_POINT('Ctrl Pts',(-0.919918268980071,0.148506890687803,
-1.02724046269848));
#46436=CARTESIAN_POINT('Ctrl Pts',(-0.879984324656564,-0.306482473469165,
-1.00753718956356));
#46437=CARTESIAN_POINT('Ctrl Pts',(-0.62863412093596,-0.68783941452938,
-0.987833916428634));
#46438=CARTESIAN_POINT('Ctrl Pts',(-0.226254551516672,-0.903942916396294,
-0.96813064329371));
#46439=CARTESIAN_POINT('Ctrl Pts',(0.23048268043472,-0.902874106509137,
-0.948427370158786));
#46440=CARTESIAN_POINT('Ctrl Pts',(0.631846441759413,-0.684889766474151,
-0.928724097023861));
#46441=CARTESIAN_POINT('Ctrl Pts',(0.881409077214873,-0.302360640276263,
-0.909020823888938));
#46442=CARTESIAN_POINT('Ctrl Pts',(0.91921315642998,0.152810638474815,-0.889317550754013));
#46443=CARTESIAN_POINT('Ctrl Pts',(0.736176248282189,0.571269156921856,
-0.86961427761909));
#46444=CARTESIAN_POINT('Ctrl Pts',(0.376272975236873,0.852480243930285,
-0.849911004484164));
#46445=CARTESIAN_POINT('Ctrl Pts',(-0.0740298909692007,0.928882927729935,
-0.830207731349242));
#46446=CARTESIAN_POINT('Ctrl Pts',(-0.506547073733252,0.782121461332782,
-0.810504458214316));
#46447=CARTESIAN_POINT('Ctrl Pts',(-0.817366307412782,0.447455291276615,
-0.790801185079393));
#46448=CARTESIAN_POINT('Ctrl Pts',(-0.931813262145332,0.00528797457665684,
-0.771097911944469));
#46449=CARTESIAN_POINT('Ctrl Pts',(-0.822392053753201,-0.438149778167965,
-0.751394638809545));
#46450=CARTESIAN_POINT('Ctrl Pts',(-0.515391130710755,-0.776322034061729,
-0.731691365674621));
#46451=CARTESIAN_POINT('Ctrl Pts',(-0.0845674736396679,-0.927982898865733,
-0.711988092539696));
#46452=CARTESIAN_POINT('Ctrl Pts',(0.366573521414127,-0.856695845433538,
-0.692284819404772));
#46453=CARTESIAN_POINT('Ctrl Pts',(0.729645217368095,-0.579587590409729,
-0.672581546269848));
#46454=CARTESIAN_POINT('Ctrl Pts',(0.917419628790013,-0.163233400061772,
-0.652878273134924));
#46455=CARTESIAN_POINT('Ctrl Pts',(0.884783947916574,0.292337619362334,
-0.633175));
#46456=CARTESIAN_POINT('Ctrl Pts',(0.639578898018757,0.677674517297069,
-0.613471726865075));
#46457=CARTESIAN_POINT('Ctrl Pts',(0.240714999413281,0.900200092892027,
-0.593768453730152));
#46458=CARTESIAN_POINT('Ctrl Pts',(-0.215980684750912,0.906452570187688,
-0.574065180595228));
#46459=CARTESIAN_POINT('Ctrl Pts',(-0.620787003165868,0.694929791333767,
-0.554361907460304));
#46460=CARTESIAN_POINT('Ctrl Pts',(-0.876449226161066,0.316450110054044,
-0.53465863432538));
#46461=CARTESIAN_POINT('Ctrl Pts',(-0.921544497258574,-0.138056719298448,
-0.514955361190455));
#46462=CARTESIAN_POINT('Ctrl Pts',(-0.745238676323796,-0.559395417857205,
-0.495252088055532));
#46463=CARTESIAN_POINT('Ctrl Pts',(-0.389889241829712,-0.84633935112569,
-0.475548814920607));
#46464=CARTESIAN_POINT('Ctrl Pts',(0.0591310941420255,-0.929950230868132,
-0.455845541785683));
#46465=CARTESIAN_POINT('Ctrl Pts',(0.493945183286743,-0.790140540785833,
-0.436142268650758));
#46466=CARTESIAN_POINT('Ctrl Pts',(0.810088927401454,-0.460499563010433,
-0.416438995515835));
#46467=CARTESIAN_POINT('Ctrl Pts',(0.931608784293944,-0.0202235518595937,
-0.39673572238091));
#46468=CARTESIAN_POINT('Ctrl Pts',(0.829309601959138,0.42491116806858,-0.377032449245987));
#46469=CARTESIAN_POINT('Ctrl Pts',(0.527768767599633,0.767960967882476,
-0.357329176111062));
#46470=CARTESIAN_POINT('Ctrl Pts',(0.0994314641129952,0.926508122447519,
-0.337625902976139));
#46471=CARTESIAN_POINT('Ctrl Pts',(-0.352794236706888,0.862461674941034,
-0.317922629841215));
#46472=CARTESIAN_POINT('Ctrl Pts',(-0.720261141223303,0.591208782986478,
-0.29821935670629));
#46473=CARTESIAN_POINT('Ctrl Pts',(-0.914685227932655,0.177917968109297,
-0.278516083571366));
#46474=CARTESIAN_POINT('Ctrl Pts',(-0.889356276613872,-0.278117652152912,
-0.258812810436442));
#46475=CARTESIAN_POINT('Ctrl Pts',(-0.650359227969422,-0.667335481823592,
-0.239109537301518));
#46476=CARTESIAN_POINT('Ctrl Pts',(-0.255113803362931,-0.896225975621676,
-0.219406264166594));
#46477=CARTESIAN_POINT('Ctrl Pts',(0.201423604491066,-0.909798087854495,
-0.19970299103167));
#46478=CARTESIAN_POINT('Ctrl Pts',(0.609567236134733,-0.704791311872434,
-0.179999717896745));
#46479=CARTESIAN_POINT('Ctrl Pts',(0.87126578132795,-0.33045814845722,-0.160296444761821));
#46480=CARTESIAN_POINT('Ctrl Pts',(0.923635855538078,0.123267091579122,
-0.140593171626897));
#46481=CARTESIAN_POINT('Ctrl Pts',(0.754115921504916,0.547378403722327,
-0.120889898491973));
#46482=CARTESIAN_POINT('Ctrl Pts',(0.403392825281099,0.839980077618579,
-0.101186625357049));
#46483=CARTESIAN_POINT('Ctrl Pts',(-0.0441920915166111,0.930780324821963,
-0.0814833522221251));
#46484=CARTESIAN_POINT('Ctrl Pts',(-0.48126923737503,0.797953792710495,
-0.0617800790872008));
#46485=CARTESIAN_POINT('Ctrl Pts',(-0.695390554538055,0.58159774764706,
-0.0486445636639179));
#46486=CARTESIAN_POINT('Ctrl Pts',(-0.770401523986372,0.454430838421997,
-0.0420768059522765));
#46487=CARTESIAN_POINT('Ctrl Pts',(-0.411771268263186,0.847217222978089,
-1.78792319404772));
#46488=CARTESIAN_POINT('Ctrl Pts',(-0.551617818839675,0.779247887686847,
-1.78135543633608));
#46489=CARTESIAN_POINT('Ctrl Pts',(-0.796874177481831,0.57280434734907,
-1.7682199209128));
#46490=CARTESIAN_POINT('Ctrl Pts',(-0.973333492885899,0.12523918821323,
-1.74851664777788));
#46491=CARTESIAN_POINT('Ctrl Pts',(-0.915933026001545,-0.352300442932758,
-1.72881337464295));
#46492=CARTESIAN_POINT('Ctrl Pts',(-0.638488140611806,-0.745255528974016,
-1.70911010150803));
#46493=CARTESIAN_POINT('Ctrl Pts',(-0.207642133040882,-0.959134995961123,
-1.6894068283731));
#46494=CARTESIAN_POINT('Ctrl Pts',(0.273087712714213,-0.942596374067765,
-1.66970355523818));
#46495=CARTESIAN_POINT('Ctrl Pts',(0.688209335308588,-0.699591806531232,
-1.65000028210326));
#46496=CARTESIAN_POINT('Ctrl Pts',(0.93798808508896,-0.288513897437003,
-1.63029700896833));
#46497=CARTESIAN_POINT('Ctrl Pts',(0.962415453602374,0.191881309378704,
-1.61059373583341));
#46498=CARTESIAN_POINT('Ctrl Pts',(0.755622338380288,0.626176102961525,
-1.59089046269848));
#46499=CARTESIAN_POINT('Ctrl Pts',(0.3672910069804,0.910032536526708,-1.57118718956356));
#46500=CARTESIAN_POINT('Ctrl Pts',(-0.109282036071534,0.975253390883418,
-1.55148391642864));
#46501=CARTESIAN_POINT('Ctrl Pts',(-0.55960004828344,0.806169709291727,
-1.53178064329371));
#46502=CARTESIAN_POINT('Ctrl Pts',(-0.875474142108766,0.443403671418404,
-1.51207737015879));
#46503=CARTESIAN_POINT('Ctrl Pts',(-0.981015543288755,-0.0258900807904488,
-1.49237409702386));
#46504=CARTESIAN_POINT('Ctrl Pts',(-0.850867934273877,-0.488963755775376,
-1.47267082388894));
#46505=CARTESIAN_POINT('Ctrl Pts',(-0.516299278280827,-0.834563866518545,
-1.45296755075401));
#46506=CARTESIAN_POINT('Ctrl Pts',(-0.057689706391535,-0.979659988189516,
-1.43326427761909));
#46507=CARTESIAN_POINT('Ctrl Pts',(0.414779819433004,-0.889392767427202,
-1.41356100448416));
#46508=CARTESIAN_POINT('Ctrl Pts',(0.787598481510704,-0.585448909629671,
-1.39385773134924));
#46509=CARTESIAN_POINT('Ctrl Pts',(0.971196585752732,-0.140850933885956,
-1.37415445821432));
#46510=CARTESIAN_POINT('Ctrl Pts',(0.921464682196681,0.337586482531115,
-1.35445118507939));
#46511=CARTESIAN_POINT('Ctrl Pts',(0.650350862167541,0.734918736907045,
-1.33474791194447));
#46512=CARTESIAN_POINT('Ctrl Pts',(0.2229902287218,0.955686743463641,-1.31504463880954));
#46513=CARTESIAN_POINT('Ctrl Pts',(-0.257943813605184,0.946850982353159,
-1.29534136567462));
#46514=CARTESIAN_POINT('Ctrl Pts',(-0.676906847271293,0.710534245387173,
-1.2756380925397));
#46515=CARTESIAN_POINT('Ctrl Pts',(-0.93324299134207,0.303511635467807,
-1.25593481940477));
#46516=CARTESIAN_POINT('Ctrl Pts',(-0.965367479808057,-0.176429653637053,
-1.23623154626985));
#46517=CARTESIAN_POINT('Ctrl Pts',(-0.765562403387109,-0.613983713361266,
-1.21652827313492));
#46518=CARTESIAN_POINT('Ctrl Pts',(-0.381830937456696,-0.904028168230564,
-1.196825));
#46519=CARTESIAN_POINT('Ctrl Pts',(0.0936354222182865,-0.976879829589592,
-1.17712172686507));
#46520=CARTESIAN_POINT('Ctrl Pts',(0.546605869002752,-0.815036083695018,
-1.15741845373015));
#46521=CARTESIAN_POINT('Ctrl Pts',(0.868254239983032,-0.457379895168767,
-1.13771518059523));
#46522=CARTESIAN_POINT('Ctrl Pts',(0.981304504747574,0.0101618263727374,
-1.1180119074603));
#46523=CARTESIAN_POINT('Ctrl Pts',(0.858596333923827,0.475262168834934,
-1.09830863432538));
#46524=CARTESIAN_POINT('Ctrl Pts',(0.529610369093823,0.826180761517367,
-1.07860536119046));
#46525=CARTESIAN_POINT('Ctrl Pts',(0.073385497803265,0.978609402399795,
-1.05890208805553));
#46526=CARTESIAN_POINT('Ctrl Pts',(-0.400470241452602,0.895927106110765,
-1.03919881492061));
#46527=CARTESIAN_POINT('Ctrl Pts',(-0.778112993640995,0.59799829672012,
-1.01949554178568));
#46528=CARTESIAN_POINT('Ctrl Pts',(-0.968814076649019,0.156400379282867,
-0.999792268650758));
#46529=CARTESIAN_POINT('Ctrl Pts',(-0.926757549779925,-0.322772733791168,
-0.980088995515835));
#46530=CARTESIAN_POINT('Ctrl Pts',(-0.662047494827864,-0.724399688255913,
-0.960385722380911));
#46531=CARTESIAN_POINT('Ctrl Pts',(-0.238280510135202,-0.951989596709347,
-0.940682449245987));
#46532=CARTESIAN_POINT('Ctrl Pts',(0.242733373994761,-0.95086397707676,
-0.920979176111061));
#46533=CARTESIAN_POINT('Ctrl Pts',(0.665430558016644,-0.721293259507376,
-0.901275902976139));
#46534=CARTESIAN_POINT('Ctrl Pts',(0.928258031269179,-0.318431815523169,
-0.881572629841214));
#46535=CARTESIAN_POINT('Ctrl Pts',(0.968071485717646,0.160932881331148,
-0.86186935670629));
#46536=CARTESIAN_POINT('Ctrl Pts',(0.775305737781691,0.601633448800766,
-0.842166083571366));
#46537=CARTESIAN_POINT('Ctrl Pts',(0.396272763966587,0.897791562831483,
-0.822462810436441));
#46538=CARTESIAN_POINT('Ctrl Pts',(-0.0779647528288262,0.978255227979619,
-0.802759537301518));
#46539=CARTESIAN_POINT('Ctrl Pts',(-0.533471235506874,0.823693046370968,
-0.783056264166593));
#46540=CARTESIAN_POINT('Ctrl Pts',(-0.860811238457195,0.471238586598027,
-0.76335299103167));
#46541=CARTESIAN_POINT('Ctrl Pts',(-0.981341316523194,0.0055690427938866,
-0.743649717896745));
#46542=CARTESIAN_POINT('Ctrl Pts',(-0.866104114970739,-0.461438463702219,
-0.723946444761821));
#46543=CARTESIAN_POINT('Ctrl Pts',(-0.542785374798827,-0.8175853659757,
-0.704243171626897));
#46544=CARTESIAN_POINT('Ctrl Pts',(-0.089062432665451,-0.977307360476132,
-0.684539898491973));
#46545=CARTESIAN_POINT('Ctrl Pts',(0.386057761486308,-0.902231233414852,
-0.664836625357049));
#46546=CARTESIAN_POINT('Ctrl Pts',(0.768427567298545,-0.610394026485191,
-0.645133352222124));
#46547=CARTESIAN_POINT('Ctrl Pts',(0.966182627888584,-0.171909637075109,
-0.625430079087201));
#46548=CARTESIAN_POINT('Ctrl Pts',(0.931812284242439,0.307876047603994,
-0.605726805952276));
#46549=CARTESIAN_POINT('Ctrl Pts',(0.673574012412253,0.71369450296019,-0.586023532817353));
#46550=CARTESIAN_POINT('Ctrl Pts',(0.253509564660249,0.948047833381428,
-0.566320259682428));
#46551=CARTESIAN_POINT('Ctrl Pts',(-0.227460563320446,0.95463264446979,
-0.546616986547504));
#46552=CARTESIAN_POINT('Ctrl Pts',(-0.65378328439402,0.731866935171721,
-0.526913713412581));
#46553=CARTESIAN_POINT('Ctrl Pts',(-0.923034552530858,0.333270173574662,
-0.507210440277655));
#46554=CARTESIAN_POINT('Ctrl Pts',(-0.970526742764244,-0.145394756841399,
-0.487507167142732));
#46555=CARTESIAN_POINT('Ctrl Pts',(-0.78484985507057,-0.589128592732363,
-0.467803894007808));
#46556=CARTESIAN_POINT('Ctrl Pts',(-0.410612766977043,-0.891324267210884,
-0.448100620872884));
#46557=CARTESIAN_POINT('Ctrl Pts',(0.0622740501022626,-0.979379260776014,
-0.428397347737959));
#46558=CARTESIAN_POINT('Ctrl Pts',(0.520199525107533,-0.832138358653435,
-0.408694074603035));
#46559=CARTESIAN_POINT('Ctrl Pts',(0.8531470486766,-0.48497619188482,-0.388990801468111));
#46560=CARTESIAN_POINT('Ctrl Pts',(0.981125970195735,-0.0212984809434644,
-0.369287528333187));
#46561=CARTESIAN_POINT('Ctrl Pts',(0.873389347043846,0.447496190511176,
-0.349584255198263));
#46562=CARTESIAN_POINT('Ctrl Pts',(0.555820912039423,0.808779889572632,
-0.329880982063339));
#46563=CARTESIAN_POINT('Ctrl Pts',(0.104716478999048,0.975754196241814,
-0.310177708928415));
#46564=CARTESIAN_POINT('Ctrl Pts',(-0.371546075567376,0.908303530246846,
-0.290474435793491));
#46565=CARTESIAN_POINT('Ctrl Pts',(-0.758544705557467,0.62263291262916,
-0.270771162658567));
#46566=CARTESIAN_POINT('Ctrl Pts',(-0.963302887229944,0.187374724261306,
-0.251067889523643));
#46567=CARTESIAN_POINT('Ctrl Pts',(-0.936627642904595,-0.292900255877137,
-0.231364616388719));
#46568=CARTESIAN_POINT('Ctrl Pts',(-0.684927342114798,-0.702805923568475,
-0.211661343253794));
#46569=CARTESIAN_POINT('Ctrl Pts',(-0.268673698718373,-0.943862482482769,
-0.19195807011887));
#46570=CARTESIAN_POINT('Ctrl Pts',(0.212129740196035,-0.958155984225694,
-0.172254796983946));
#46571=CARTESIAN_POINT('Ctrl Pts',(0.641967160502342,-0.742252618592942,
-0.152551523849022));
#46572=CARTESIAN_POINT('Ctrl Pts',(0.917575595480876,-0.348022771983522,
-0.132848250714098));
#46573=CARTESIAN_POINT('Ctrl Pts',(0.972729261627955,0.129819025816112,
-0.113144977579174));
#46574=CARTESIAN_POINT('Ctrl Pts',(0.794198946596785,0.57647284618863,-0.0934417044442497));
#46575=CARTESIAN_POINT('Ctrl Pts',(0.424834097473517,0.884626983442641,
-0.0737384313093252));
#46576=CARTESIAN_POINT('Ctrl Pts',(-0.046541004545243,0.980253476165065,
-0.0540351581744016));
#46577=CARTESIAN_POINT('Ctrl Pts',(-0.506849823021797,0.840366903192951,
-0.0343318850394773));
#46578=CARTESIAN_POINT('Ctrl Pts',(-0.732352189018033,0.612511028281409,
-0.0211963696161944));
#46579=CARTESIAN_POINT('Ctrl Pts',(-0.811350166941868,0.478584900389869,
-0.014628611904553));
#46580=CARTESIAN_POINT('Ctrl Pts',(-0.432553262684897,0.889976067411731,
-1.760475));
#46581=CARTESIAN_POINT('Ctrl Pts',(-0.579457834201591,0.818576336520457,
-1.75390724228836));
#46582=CARTESIAN_POINT('Ctrl Pts',(-0.837092220817113,0.601713641583103,
-1.74077172686507));
#46583=CARTESIAN_POINT('Ctrl Pts',(-1.02245739437844,0.131559979175176,
-1.72106845373015));
#46584=CARTESIAN_POINT('Ctrl Pts',(-0.962159940077686,-0.370080959457566,
-1.70136518059523));
#46585=CARTESIAN_POINT('Ctrl Pts',(-0.670712479703,-0.782868391841341,-1.6816619074603));
#46586=CARTESIAN_POINT('Ctrl Pts',(-0.218121780318774,-1.00754230281332,
-1.66195863432538));
#46587=CARTESIAN_POINT('Ctrl Pts',(0.28687038226812,-0.990168980749204,
-1.64225536119046));
#46588=CARTESIAN_POINT('Ctrl Pts',(0.722943090841553,-0.734900032581417,
-1.62255208805553));
#46589=CARTESIAN_POINT('Ctrl Pts',(0.985328112561426,-0.303075122731843,
-1.60284881492061));
#46590=CARTESIAN_POINT('Ctrl Pts',(1.0109883243432,0.201565511770867,-1.58314554178568));
#46591=CARTESIAN_POINT('Ctrl Pts',(0.793758411563286,0.657779056547004,
-1.56344226865076));
#46592=CARTESIAN_POINT('Ctrl Pts',(0.385828093578033,0.955961654353322,
-1.54373899551583));
#46593=CARTESIAN_POINT('Ctrl Pts',(-0.11479747349778,1.02447418915471,-1.52403572238091));
#46594=CARTESIAN_POINT('Ctrl Pts',(-0.587842924798037,0.846856895826426,
-1.50433244924599));
#46595=CARTESIAN_POINT('Ctrl Pts',(-0.919659106286569,0.465782145431056,
-1.48462917611106));
#46596=CARTESIAN_POINT('Ctrl Pts',(-1.03052715597177,-0.0271967467869228,
-1.46492590297614));
#46597=CARTESIAN_POINT('Ctrl Pts',(-0.893811029206843,-0.51364163601652,
-1.44522262984121));
#46598=CARTESIAN_POINT('Ctrl Pts',(-0.542356775605552,-0.876684099170293,
-1.42551935670629));
#46599=CARTESIAN_POINT('Ctrl Pts',(-0.0606012916545775,-1.02910318634077,
-1.40581608357137));
#46600=CARTESIAN_POINT('Ctrl Pts',(0.435713654690751,-0.934280201194361,
-1.38611281043644));
#46601=CARTESIAN_POINT('Ctrl Pts',(0.827348382756466,-0.614996371805552,
-1.36640953730152));
#46602=CARTESIAN_POINT('Ctrl Pts',(1.02021263806894,-0.147959645804244,
-1.34670626416659));
#46603=CARTESIAN_POINT('Ctrl Pts',(0.967970777597627,0.354624389100941,
-1.32700299103167));
#46604=CARTESIAN_POINT('Ctrl Pts',(0.683173909891899,0.772009904426415,
-1.30729971789675));
#46605=CARTESIAN_POINT('Ctrl Pts',(0.234244490605928,1.00392001786216,-1.28759644476182));
#46606=CARTESIAN_POINT('Ctrl Pts',(-0.270962174303511,0.994638318066147,
-1.2678931716269));
#46607=CARTESIAN_POINT('Ctrl Pts',(-0.711070169018694,0.746394733629479,
-1.24818989849197));
#46608=CARTESIAN_POINT('Ctrl Pts',(-0.980343535102633,0.318829792904634,
-1.22848662535705));
#46609=CARTESIAN_POINT('Ctrl Pts',(-1.01408933858391,-0.185334014772241,
-1.20878335222212));
#46610=CARTESIAN_POINT('Ctrl Pts',(-0.804200149201113,-0.644971320048627,
-1.1890800790872));
#46611=CARTESIAN_POINT('Ctrl Pts',(-0.401101850761873,-0.949654247069143,
-1.16937680595228));
#46612=CARTESIAN_POINT('Ctrl Pts',(0.0983611788997142,-1.02618271382152,
-1.14967353281735));
#46613=CARTESIAN_POINT('Ctrl Pts',(0.574192932491672,-0.856170753960593,
-1.12997025968243));
#46614=CARTESIAN_POINT('Ctrl Pts',(0.912074817480007,-0.480463745749438,
-1.1102669865475));
#46615=CARTESIAN_POINT('Ctrl Pts',(1.03083070124419,0.0106746912452258,
-1.09056371341258));
#46616=CARTESIAN_POINT('Ctrl Pts',(0.901929479282339,0.499248533360167,
-1.07086044027766));
#46617=CARTESIAN_POINT('Ctrl Pts',(0.55633967389115,0.867877900925852,-1.05115716714273));
#46618=CARTESIAN_POINT('Ctrl Pts',(0.0770892457903824,1.02799957774517,
-1.03145389400781));
#46619=CARTESIAN_POINT('Ctrl Pts',(-0.4206818758365,0.941144326340793,-1.01175062087288));
#46620=CARTESIAN_POINT('Ctrl Pts',(-0.817384164651821,0.628179123369462,
-0.992047347737959));
#46621=CARTESIAN_POINT('Ctrl Pts',(-1.01770988431797,0.164293867877931,
-0.972344074603035));
#46622=CARTESIAN_POINT('Ctrl Pts',(-0.973530774903286,-0.339062994113169,
-0.952640801468111));
#46623=CARTESIAN_POINT('Ctrl Pts',(-0.695460868719769,-0.760959961982448,
-0.932937528333187));
#46624=CARTESIAN_POINT('Ctrl Pts',(-0.250306468753732,-1.0000362770224,
-0.913234255198262));
#46625=CARTESIAN_POINT('Ctrl Pts',(0.254984067554803,-0.998853847644383,
-0.89353098206334));
#46626=CARTESIAN_POINT('Ctrl Pts',(0.699014674273875,-0.7576967525406,-0.873827708928414));
#46627=CARTESIAN_POINT('Ctrl Pts',(0.975106985323486,-0.334502990770076,
-0.854124435793491));
#46628=CARTESIAN_POINT('Ctrl Pts',(1.01692981500531,0.16905512418748,-0.834421162658567));
#46629=CARTESIAN_POINT('Ctrl Pts',(0.814435227281192,0.631997740679676,
-0.814717889523642));
#46630=CARTESIAN_POINT('Ctrl Pts',(0.416272552696301,0.94310288173268,-0.795014616388719));
#46631=CARTESIAN_POINT('Ctrl Pts',(-0.0818996146884514,1.0276275282293,
-0.775311343253793));
#46632=CARTESIAN_POINT('Ctrl Pts',(-0.560395397280496,0.865264631409154,
-0.755608070118871));
#46633=CARTESIAN_POINT('Ctrl Pts',(-0.904256169501606,0.495021881919439,
-0.735904796983944));
#46634=CARTESIAN_POINT('Ctrl Pts',(-1.03086937090106,0.00585011101111694,
-0.716201523849023));
#46635=CARTESIAN_POINT('Ctrl Pts',(-0.909816176188277,-0.484727149236474,
-0.696498250714097));
#46636=CARTESIAN_POINT('Ctrl Pts',(-0.570179618886898,-0.858848697889669,
-0.676794977579175));
#46637=CARTESIAN_POINT('Ctrl Pts',(-0.0935573916912343,-1.02663182208653,
-0.657091704444248));
#46638=CARTESIAN_POINT('Ctrl Pts',(0.40554200155849,-0.947766621396166,
-0.637388431309326));
#46639=CARTESIAN_POINT('Ctrl Pts',(0.807209917228995,-0.641200462560654,
-0.617685158174401));
#46640=CARTESIAN_POINT('Ctrl Pts',(1.01494562698716,-0.180585874088446,
-0.597981885039478));
#46641=CARTESIAN_POINT('Ctrl Pts',(0.978840620568303,0.323414475845652,
-0.578278611904553));
#46642=CARTESIAN_POINT('Ctrl Pts',(0.707569126805749,0.749714488623311,
-0.55857533876963));
#46643=CARTESIAN_POINT('Ctrl Pts',(0.266304129907217,0.99589557387083,-0.538872065634705));
#46644=CARTESIAN_POINT('Ctrl Pts',(-0.238940441889981,1.00281271875189,
-0.519168792499781));
#46645=CARTESIAN_POINT('Ctrl Pts',(-0.686779565622172,0.768804079009677,
-0.499465519364857));
#46646=CARTESIAN_POINT('Ctrl Pts',(-0.969619878900649,0.350090237095279,
-0.479762246229933));
#46647=CARTESIAN_POINT('Ctrl Pts',(-1.01950898826992,-0.152732794384349,
-0.460058973095008));
#46648=CARTESIAN_POINT('Ctrl Pts',(-0.824461033817341,-0.618861767607521,
-0.440355699960084));
#46649=CARTESIAN_POINT('Ctrl Pts',(-0.431336292124375,-0.936309183296075,
-0.42065242682516));
#46650=CARTESIAN_POINT('Ctrl Pts',(0.0654170060624995,-1.0288082906839,
-0.400949153690236));
#46651=CARTESIAN_POINT('Ctrl Pts',(0.546453866928323,-0.874136176521035,
-0.381245880555312));
#46652=CARTESIAN_POINT('Ctrl Pts',(0.896205169951745,-0.509452820759208,
-0.361542607420388));
#46653=CARTESIAN_POINT('Ctrl Pts',(1.03064315609753,-0.0223734100273349,
-0.341839334285463));
#46654=CARTESIAN_POINT('Ctrl Pts',(0.917469092128553,0.470081212953772,
-0.32213606115054));
#46655=CARTESIAN_POINT('Ctrl Pts',(0.583873056479214,0.849598811262788,
-0.302432788015615));
#46656=CARTESIAN_POINT('Ctrl Pts',(0.110001493885101,1.02500027003611,-0.282729514880691));
#46657=CARTESIAN_POINT('Ctrl Pts',(-0.390297914427862,0.954145385552656,
-0.263026241745767));
#46658=CARTESIAN_POINT('Ctrl Pts',(-0.796828269891632,0.654057042271841,
-0.243322968610843));
#46659=CARTESIAN_POINT('Ctrl Pts',(-1.01192054652723,0.196831480413315,
-0.223619695475919));
#46660=CARTESIAN_POINT('Ctrl Pts',(-0.983899009195318,-0.307682859601362,
-0.203916422340995));
#46661=CARTESIAN_POINT('Ctrl Pts',(-0.719495456260174,-0.738276365313358,
-0.184213149206071));
#46662=CARTESIAN_POINT('Ctrl Pts',(-0.282233594073814,-0.991498989343861,
-0.164509876071147));
#46663=CARTESIAN_POINT('Ctrl Pts',(0.222835875901004,-1.00651388059689,
-0.144806602936223));
#46664=CARTESIAN_POINT('Ctrl Pts',(0.674367084869952,-0.779713925313451,
-0.125103329801299));
#46665=CARTESIAN_POINT('Ctrl Pts',(0.963885409633801,-0.365587395509823,
-0.105400056666374));
#46666=CARTESIAN_POINT('Ctrl Pts',(1.02182266771783,0.136370960053101,-0.0856967835314503));
#46667=CARTESIAN_POINT('Ctrl Pts',(0.834281971688654,0.605567288654934,
-0.0659935103965262));
#46668=CARTESIAN_POINT('Ctrl Pts',(0.446275369665935,0.929273889266702,
-0.0462902372616017));
#46669=CARTESIAN_POINT('Ctrl Pts',(-0.0488899175738751,1.02972662750817,
-0.0265869641266781));
#46670=CARTESIAN_POINT('Ctrl Pts',(-0.532430408668564,0.882780013675407,
-0.00688369099175381));
#46671=CARTESIAN_POINT('Ctrl Pts',(-0.769313823498012,0.643424308915757,
0.0062518244315291));
#46672=CARTESIAN_POINT('Ctrl Pts',(-0.852298809897364,0.502738962357741,
0.0128195821431705));
#46673=CARTESIAN_POINT('Ctrl Pts',(-0.989459186063674,1.54013734824731E-5,
-0.215975728002209));
#46674=CARTESIAN_POINT('Ctrl Pts',(-0.98940307000832,-0.0999713176614304,
-0.211955959448471));
#46675=CARTESIAN_POINT('Ctrl Pts',(-0.974331598209586,-0.199974581563408,
-0.207936190894733));
#46676=CARTESIAN_POINT('Ctrl Pts',(-0.94450200659478,-0.295362720550915,
-0.203916422340995));
#46677=CARTESIAN_POINT('Ctrl Pts',(-0.89576449155027,-0.451214028172027,
-0.197348664629354));
#46678=CARTESIAN_POINT('Ctrl Pts',(-0.807629973905222,-0.594745196742693,
-0.190780906917712));
#46679=CARTESIAN_POINT('Ctrl Pts',(-0.690685738051638,-0.708714551699776,
-0.184213149206071));
#46680=CARTESIAN_POINT('Ctrl Pts',(-0.573741502198054,-0.822683906656859,
-0.177645391494429));
#46681=CARTESIAN_POINT('Ctrl Pts',(-0.427987548135934,-0.90709144800036,
-0.171077633782788));
#46682=CARTESIAN_POINT('Ctrl Pts',(-0.270932326109071,-0.951797700547616,
-0.164509876071147));
#46683=CARTESIAN_POINT('Ctrl Pts',(-0.113877104082208,-0.996503953094872,
-0.157942118359506));
#46684=CARTESIAN_POINT('Ctrl Pts',(0.0544793859093978,-1.00150891684588,
-0.151374360647864));
#46685=CARTESIAN_POINT('Ctrl Pts',(0.213912832400026,-0.966211406174147,
-0.144806602936223));
#46686=CARTESIAN_POINT('Ctrl Pts',(0.373346278890653,-0.930913895502412,
-0.138238845224581));
#46687=CARTESIAN_POINT('Ctrl Pts',(0.523856681880303,-0.855313910407931,
-0.13167108751294));
#46688=CARTESIAN_POINT('Ctrl Pts',(0.647364937502435,-0.748492829560086,
-0.125103329801298));
#46689=CARTESIAN_POINT('Ctrl Pts',(0.770873193124568,-0.641671748712241,
-0.118535572089657));
#46690=CARTESIAN_POINT('Ctrl Pts',(0.867379301379184,-0.503629572111032,
-0.111967814378016));
#46691=CARTESIAN_POINT('Ctrl Pts',(0.925288565187164,-0.350948757883274,
-0.105400056666374));
#46692=CARTESIAN_POINT('Ctrl Pts',(0.983197828995144,-0.198267943655515,
-0.0988322989547328));
#46693=CARTESIAN_POINT('Ctrl Pts',(1.00251024835649,-0.0309484918012002,
-0.0922645412430913));
#46694=CARTESIAN_POINT('Ctrl Pts',(0.980909675365629,0.13091062222626,-0.08569678353145));
#46695=CARTESIAN_POINT('Ctrl Pts',(0.963180651960666,0.263759136111232,
-0.0803061890209666));
#46696=CARTESIAN_POINT('Ctrl Pts',(0.917890288593679,0.392929253024943,
-0.0749155945104836));
#46697=CARTESIAN_POINT('Ctrl Pts',(0.849186560444991,0.508032827447782,
-0.0695250000000002));
#46698=CARTESIAN_POINT('',(-0.491859688152273,-0.689459403554686,-1.760475));
#46699=CARTESIAN_POINT('Ctrl Pts',(-0.491859688152275,-0.689459403554684,
-1.760475));
#46700=CARTESIAN_POINT('Ctrl Pts',(-0.513554842694071,-0.676529705956258,
-1.760475));
#46701=CARTESIAN_POINT('Ctrl Pts',(-0.534635231361505,-0.662644680299156,
-1.760475));
#46702=CARTESIAN_POINT('Ctrl Pts',(-0.555033286604471,-0.647841975554216,
-1.760475));
#46703=CARTESIAN_POINT('Ctrl Pts',(-0.58415798250627,-0.626706417821615,
-1.760475));
#46704=CARTESIAN_POINT('Ctrl Pts',(-0.611892735613209,-0.603701443225965,
-1.760475));
#46705=CARTESIAN_POINT('Ctrl Pts',(-0.638121657096046,-0.579014067915186,
-1.760475));
#46706=CARTESIAN_POINT('Ctrl Pts',(-0.646098901072591,-0.571505668604011,
-1.760475));
#46707=CARTESIAN_POINT('Ctrl Pts',(-0.65393672584828,-0.563841411402002,
-1.760475));
#46708=CARTESIAN_POINT('Ctrl Pts',(-0.661631495607065,-0.556025978619957,
-1.760475));
#46709=CARTESIAN_POINT('Ctrl Pts',(-0.668300148268516,-0.549252753655965,
-1.760475));
#46710=CARTESIAN_POINT('Ctrl Pts',(-0.674859642024538,-0.54236754289441,
-1.760475));
#46711=CARTESIAN_POINT('Ctrl Pts',(-0.681300291911483,-0.535381927138061,
-1.760475));
#46712=CARTESIAN_POINT('Ctrl Pts',(-0.708273869420477,-0.506126021078973,
-1.760475));
#46713=CARTESIAN_POINT('Ctrl Pts',(-0.733203917913654,-0.475073691031234,
-1.760475));
#46714=CARTESIAN_POINT('Ctrl Pts',(-0.755936918937743,-0.442469540470751,
-1.760475));
#46715=CARTESIAN_POINT('Ctrl Pts',(-0.77218026589336,-0.419172988942604,
-1.760475));
#46716=CARTESIAN_POINT('Ctrl Pts',(-0.78730146906442,-0.395083087809655,
-1.760475));
#46717=CARTESIAN_POINT('Ctrl Pts',(-0.801233694577352,-0.370277201526068,
-1.760475));
#46718=CARTESIAN_POINT('Ctrl Pts',(-0.805786257659718,-0.362171507140401,
-1.760475));
#46719=CARTESIAN_POINT('Ctrl Pts',(-0.810207227008384,-0.353997321790457,
-1.760475));
#46720=CARTESIAN_POINT('Ctrl Pts',(-0.814493086153977,-0.345761134855412,
-1.760475));
#46721=CARTESIAN_POINT('Ctrl Pts',(-0.819180750550855,-0.336752793948747,
-1.760475));
#46722=CARTESIAN_POINT('Ctrl Pts',(-0.823707501249501,-0.327669012074212,
-1.760475));
#46723=CARTESIAN_POINT('Ctrl Pts',(-0.828071044204866,-0.318513817684205,
-1.760475));
#46724=CARTESIAN_POINT('Ctrl Pts',(-0.845392775283347,-0.282170915410279,
-1.760475));
#46725=CARTESIAN_POINT('Ctrl Pts',(-0.860145988846534,-0.244705464421566,
-1.760475));
#46726=CARTESIAN_POINT('Ctrl Pts',(-0.872333447502791,-0.206410510016498,
-1.760475));
#46727=CARTESIAN_POINT('Ctrl Pts',(-0.881034937585783,-0.179069029287595,
-1.760475));
#46728=CARTESIAN_POINT('Ctrl Pts',(-0.888427703296585,-0.151303781793152,
-1.760475));
#46729=CARTESIAN_POINT('Ctrl Pts',(-0.894498914094688,-0.12321284647818,
-1.760475));
#46730=CARTESIAN_POINT('Ctrl Pts',(-0.89903476223958,-0.102225893286487,
-1.760475));
#46731=CARTESIAN_POINT('Ctrl Pts',(-0.902832725396058,-0.0810569930890353,
-1.760475));
#46732=CARTESIAN_POINT('Ctrl Pts',(-0.905882898683675,-0.0597456113193039,
-1.760475));
#46733=CARTESIAN_POINT('Ctrl Pts',(-0.907009065019949,-0.0518771532136601,
-1.760475));
#46734=CARTESIAN_POINT('Ctrl Pts',(-0.9080335392552,-0.0439867555116406,
-1.760475));
#46735=CARTESIAN_POINT('Ctrl Pts',(-0.908954731322743,-0.0360847177437703,
-1.760475));
#46736=CARTESIAN_POINT('Ctrl Pts',(-0.913760013494143,0.00513526508232103,
-1.760475));
#46737=CARTESIAN_POINT('Ctrl Pts',(-0.915746617672292,0.0465497049188463,
-1.760475));
#46738=CARTESIAN_POINT('Ctrl Pts',(-0.914906895042617,0.0878627812257661,
-1.760475));
#46739=CARTESIAN_POINT('Ctrl Pts',(-0.914705277088933,0.0977820779209303,
-1.760475));
#46740=CARTESIAN_POINT('Ctrl Pts',(-0.914340512210413,0.107695632494892,
-1.760475));
#46741=CARTESIAN_POINT('Ctrl Pts',(-0.913812080888137,0.117599511663197,
-1.760475));
#46742=CARTESIAN_POINT('Ctrl Pts',(-0.911747207846467,0.156299437728377,
-1.760475));
#46743=CARTESIAN_POINT('Ctrl Pts',(-0.90718655399813,0.194851447623349,
-1.760475));
#46744=CARTESIAN_POINT('Ctrl Pts',(-0.900223938978484,0.233041812511025,
-1.760475));
#46745=CARTESIAN_POINT('Ctrl Pts',(-0.896568758292669,0.253090699851166,
-1.760475));
#46746=CARTESIAN_POINT('Ctrl Pts',(-0.892250917284448,0.273039973286555,
-1.760475));
#46747=CARTESIAN_POINT('Ctrl Pts',(-0.887279551691811,0.292858392455839,
-1.760475));
#46748=CARTESIAN_POINT('Ctrl Pts',(-0.885185218028628,0.301207483192346,
-1.760475));
#46749=CARTESIAN_POINT('Ctrl Pts',(-0.882974289057405,0.30953537751547,
-1.760475));
#46750=CARTESIAN_POINT('Ctrl Pts',(-0.880649122486369,0.317833204271337,
-1.760475));
#46751=CARTESIAN_POINT('Ctrl Pts',(-0.868801101037989,0.36011526294322,
-1.760475));
#46752=CARTESIAN_POINT('Ctrl Pts',(-0.854043141892115,0.401439171484018,
-1.760475));
#46753=CARTESIAN_POINT('Ctrl Pts',(-0.836535505825568,0.441508132758752,
-1.760475));
#46754=CARTESIAN_POINT('Ctrl Pts',(-0.819027869759021,0.481577094033486,
-1.760475));
#46755=CARTESIAN_POINT('Ctrl Pts',(-0.798770224193348,0.520392501962671,
-1.760475));
#46756=CARTESIAN_POINT('Ctrl Pts',(-0.775863758341581,0.557650930856443,
-1.760475));
#46757=CARTESIAN_POINT('Ctrl Pts',(-0.765346338316838,0.574758002225448,
-1.760475));
#46758=CARTESIAN_POINT('Ctrl Pts',(-0.754269712559982,0.591536614134397,
-1.760475));
#46759=CARTESIAN_POINT('Ctrl Pts',(-0.742655654021007,0.607967592002281,
-1.760475));
#46760=CARTESIAN_POINT('Ctrl Pts',(-0.735908143868069,0.617513625338877,
-1.760475));
#46761=CARTESIAN_POINT('Ctrl Pts',(-0.728979187640245,0.626942295282531,
-1.760475));
#46762=CARTESIAN_POINT('Ctrl Pts',(-0.721872716760233,0.636249606571553,
-1.760475));
#46763=CARTESIAN_POINT('Ctrl Pts',(-0.716795469419606,0.642899253391818,
-1.760475));
#46764=CARTESIAN_POINT('Ctrl Pts',(-0.71162765235188,0.649486685668207,
-1.760475));
#46765=CARTESIAN_POINT('Ctrl Pts',(-0.706379814108373,0.655999601780021,
-1.760475));
#46766=CARTESIAN_POINT('Ctrl Pts',(-0.679428641377427,0.68944779872642,
-1.760475));
#46767=CARTESIAN_POINT('Ctrl Pts',(-0.65031445627706,0.721007357869669,
-1.760475));
#46768=CARTESIAN_POINT('Ctrl Pts',(-0.619290562197985,0.750520252800286,
-1.760475));
#46769=CARTESIAN_POINT('Ctrl Pts',(-0.587986290776079,0.780299869472499,
-1.760475));
#46770=CARTESIAN_POINT('Ctrl Pts',(-0.554736927205615,0.807996564025384,
-1.760475));
#46771=CARTESIAN_POINT('Ctrl Pts',(-0.519757449609006,0.833421359243327,
-1.760475));
#46772=CARTESIAN_POINT('Ctrl Pts',(-0.491766816907548,0.853766320156187,
-1.760475));
#46773=CARTESIAN_POINT('Ctrl Pts',(-0.462667324820022,0.872656204698553,
-1.760475));
#46774=CARTESIAN_POINT('Ctrl Pts',(-0.4325532626849,0.88997606741173,-1.760475));
#46775=CARTESIAN_POINT('Ctrl Pts',(-0.491859688152273,-0.689459403554686,
-1.760475));
#46776=CARTESIAN_POINT('Ctrl Pts',(-0.398395568260706,-0.755994133601717,
-1.75508440548952));
#46777=CARTESIAN_POINT('Ctrl Pts',(-0.16086093226988,-0.861432027295567,
-1.74312605326739));
#46778=CARTESIAN_POINT('Ctrl Pts',(0.2455223736064,-0.847451160704884,-1.72459994333363));
#46779=CARTESIAN_POINT('Ctrl Pts',(0.618741824242655,-0.628975354430863,
-1.7048966701987));
#46780=CARTESIAN_POINT('Ctrl Pts',(0.843308030144031,-0.259391446847321,
-1.68519339706378));
#46781=CARTESIAN_POINT('Ctrl Pts',(0.865269712120719,0.172512904594376,
-1.66549012392885));
#46782=CARTESIAN_POINT('Ctrl Pts',(0.679350192014294,0.562970195790566,
-1.64578685079393));
#46783=CARTESIAN_POINT('Ctrl Pts',(0.330216833785133,0.818174300873478,
-1.626083577659));
#46784=CARTESIAN_POINT('Ctrl Pts',(-0.0982511612190419,0.876811794340843,
-1.60638030452408));
#46785=CARTESIAN_POINT('Ctrl Pts',(-0.503114295254248,0.724795336222326,
-1.58667703138916));
#46786=CARTESIAN_POINT('Ctrl Pts',(-0.782060386406126,0.404439313852934,
-1.56732369992959));
#46787=CARTESIAN_POINT('Ctrl Pts',(-0.846902938248956,0.132306308151429,
-1.55453812618166));
#46788=CARTESIAN_POINT('Ctrl Pts',(-0.846965023971566,-7.48627396995969E-6,
-1.54832031014538));
#46789=CARTESIAN_POINT('Origin',(-9.02152032747242E-17,0.,-1.760475));
#46790=CARTESIAN_POINT('',(-0.989525,-1.21181862392629E-16,-1.760475));
#46791=CARTESIAN_POINT('Origin',(0.,0.,-1.760475));
#46792=CARTESIAN_POINT('Origin',(0.,0.,-1.760475));
#46793=CARTESIAN_POINT('',(0.4918304658226,-0.689450798018774,-1.760475));
#46794=CARTESIAN_POINT('Ctrl Pts',(0.432585265653203,0.889991656643918,
-1.760475));
#46795=CARTESIAN_POINT('Ctrl Pts',(0.45798591835325,0.875415629978971,-1.760475));
#46796=CARTESIAN_POINT('Ctrl Pts',(0.482694780440998,0.859730461206841,
-1.760475));
#46797=CARTESIAN_POINT('Ctrl Pts',(0.506629023856996,0.84296098228689,-1.760475));
#46798=CARTESIAN_POINT('Ctrl Pts',(0.53935338136335,0.820032727825965,-1.760475));
#46799=CARTESIAN_POINT('Ctrl Pts',(0.570631005944284,0.795078082524571,
-1.760475));
#46800=CARTESIAN_POINT('Ctrl Pts',(0.600302577473977,0.768263021275726,
-1.760475));
#46801=CARTESIAN_POINT('Ctrl Pts',(0.610454158722013,0.759088742364806,
-1.760475));
#46802=CARTESIAN_POINT('Ctrl Pts',(0.620417490178586,0.749696503061233,
-1.760475));
#46803=CARTESIAN_POINT('Ctrl Pts',(0.630185343180822,0.740092423589821,
-1.760475));
#46804=CARTESIAN_POINT('Ctrl Pts',(0.637344475756988,0.733053325213531,
-1.760475));
#46805=CARTESIAN_POINT('Ctrl Pts',(0.644397060752394,0.725901766656863,
-1.760475));
#46806=CARTESIAN_POINT('Ctrl Pts',(0.651332664052404,0.718648627745557,
-1.760475));
#46807=CARTESIAN_POINT('Ctrl Pts',(0.681005868927243,0.687616882187022,
-1.760475));
#46808=CARTESIAN_POINT('Ctrl Pts',(0.708583107655331,0.654687253158885,
-1.760475));
#46809=CARTESIAN_POINT('Ctrl Pts',(0.733863523204194,0.620067867414038,
-1.760475));
#46810=CARTESIAN_POINT('Ctrl Pts',(0.751151766686191,0.596393083714486,
-1.760475));
#46811=CARTESIAN_POINT('Ctrl Pts',(0.767365051485111,0.571927361560537,
-1.760475));
#46812=CARTESIAN_POINT('Ctrl Pts',(0.782425995121837,0.546731616997909,
-1.760475));
#46813=CARTESIAN_POINT('Ctrl Pts',(0.787284585117823,0.538603587611031,
-1.760475));
#46814=CARTESIAN_POINT('Ctrl Pts',(0.792023989005052,0.530397840115069,
-1.760475));
#46815=CARTESIAN_POINT('Ctrl Pts',(0.796633225077183,0.522131632421258,
-1.760475));
#46816=CARTESIAN_POINT('Ctrl Pts',(0.803720470973657,0.509421359907429,
-1.760475));
#46817=CARTESIAN_POINT('Ctrl Pts',(0.810504546411578,0.496560849854548,
-1.760475));
#46818=CARTESIAN_POINT('Ctrl Pts',(0.816978165074221,0.483558434025041,
-1.760475));
#46819=CARTESIAN_POINT('Ctrl Pts',(0.835762792526234,0.445829066562774,
-1.760475));
#46820=CARTESIAN_POINT('Ctrl Pts',(0.851937120041244,0.406905973470094,
-1.760475));
#46821=CARTESIAN_POINT('Ctrl Pts',(0.865448139529281,0.367072134072767,
-1.760475));
#46822=CARTESIAN_POINT('Ctrl Pts',(0.878840701435135,0.327587537033374,
-1.760475));
#46823=CARTESIAN_POINT('Ctrl Pts',(0.889616537975764,0.287206908970188,
-1.760475));
#46824=CARTESIAN_POINT('Ctrl Pts',(0.89767373544074,0.246200579867532,-1.760475));
#46825=CARTESIAN_POINT('Ctrl Pts',(0.901076744052898,0.228881295873818,
-1.760475));
#46826=CARTESIAN_POINT('Ctrl Pts',(0.903994163014496,0.211450433808179,
-1.760475));
#46827=CARTESIAN_POINT('Ctrl Pts',(0.906415520733311,0.193928848146053,
-1.760475));
#46828=CARTESIAN_POINT('Ctrl Pts',(0.907539225087183,0.185797425869091,
-1.760475));
#46829=CARTESIAN_POINT('Ctrl Pts',(0.908554772027421,0.177655725181455,
-1.760475));
#46830=CARTESIAN_POINT('Ctrl Pts',(0.909461566888417,0.169507887069413,
-1.760475));
#46831=CARTESIAN_POINT('Ctrl Pts',(0.914011444452751,0.128625800703072,
-1.760475));
#46832=CARTESIAN_POINT('Ctrl Pts',(0.915829911660294,0.0875722848076394,
-1.760475));
#46833=CARTESIAN_POINT('Ctrl Pts',(0.914846868041438,0.046609243460652,
-1.760475));
#46834=CARTESIAN_POINT('Ctrl Pts',(0.914761251370463,0.0430416304210539,
-1.760475));
#46835=CARTESIAN_POINT('Ctrl Pts',(0.91465435174813,0.0394747054990269,
-1.760475));
#46836=CARTESIAN_POINT('Ctrl Pts',(0.914526104044267,0.0359086435694835,
-1.760475));
#46837=CARTESIAN_POINT('Ctrl Pts',(0.913191646411139,-0.0011973506802701,
-1.760475));
#46838=CARTESIAN_POINT('Ctrl Pts',(0.909548495924747,-0.0382108997772076,
-1.760475));
#46839=CARTESIAN_POINT('Ctrl Pts',(0.903640101856299,-0.074922457480337,
-1.760475));
#46840=CARTESIAN_POINT('Ctrl Pts',(0.900537698662256,-0.0941991090640101,
-1.760475));
#46841=CARTESIAN_POINT('Ctrl Pts',(0.89681019627246,-0.113392304066952,
-1.760475));
#46842=CARTESIAN_POINT('Ctrl Pts',(0.89246049865831,-0.132469853078937,
-1.760475));
#46843=CARTESIAN_POINT('Ctrl Pts',(0.890507239189318,-0.141036748196337,
-1.760475));
#46844=CARTESIAN_POINT('Ctrl Pts',(0.888428483231742,-0.149580301912525,
-1.760475));
#46845=CARTESIAN_POINT('Ctrl Pts',(0.886224351701397,-0.158097485205295,
-1.760475));
#46846=CARTESIAN_POINT('Ctrl Pts',(0.884233674210441,-0.165789841507014,
-1.760475));
#46847=CARTESIAN_POINT('Ctrl Pts',(0.882143031893133,-0.173451728693595,
-1.760475));
#46848=CARTESIAN_POINT('Ctrl Pts',(0.879953614149768,-0.181079610448173,
-1.760475));
#46849=CARTESIAN_POINT('Ctrl Pts',(0.868866441708987,-0.219707067737752,
-1.760475));
#46850=CARTESIAN_POINT('Ctrl Pts',(0.855246588377019,-0.257477541532766,
-1.760475));
#46851=CARTESIAN_POINT('Ctrl Pts',(0.839165814934115,-0.294129295903733,
-1.760475));
#46852=CARTESIAN_POINT('Ctrl Pts',(0.82503338612271,-0.326340327997428,
-1.760475));
#46853=CARTESIAN_POINT('Ctrl Pts',(0.808999319325282,-0.357687581877215,
-1.760475));
#46854=CARTESIAN_POINT('Ctrl Pts',(0.79108449509014,-0.387975132360534,
-1.760475));
#46855=CARTESIAN_POINT('Ctrl Pts',(0.781747975332567,-0.403759842820672,
-1.760475));
#46856=CARTESIAN_POINT('Ctrl Pts',(0.771900190824228,-0.419256373417897,
-1.760475));
#46857=CARTESIAN_POINT('Ctrl Pts',(0.761557518747048,-0.434442544451675,
-1.760475));
#46858=CARTESIAN_POINT('Ctrl Pts',(0.754293562385933,-0.445108229572368,
-1.760475));
#46859=CARTESIAN_POINT('Ctrl Pts',(0.746785465653178,-0.45562078837041,
-1.760475));
#46860=CARTESIAN_POINT('Ctrl Pts',(0.739038567160396,-0.465971948253785,
-1.760475));
#46861=CARTESIAN_POINT('Ctrl Pts',(0.734132940351708,-0.472526691093413,
-1.760475));
#46862=CARTESIAN_POINT('Ctrl Pts',(0.729136752700646,-0.479009696834791,
-1.760475));
#46863=CARTESIAN_POINT('Ctrl Pts',(0.724054279914929,-0.485416368873636,
-1.760475));
#46864=CARTESIAN_POINT('Ctrl Pts',(0.699539728324438,-0.516317998619886,
-1.760475));
#46865=CARTESIAN_POINT('Ctrl Pts',(0.673003337176752,-0.545469980344396,
-1.760475));
#46866=CARTESIAN_POINT('Ctrl Pts',(0.644641319797155,-0.572683000469787,
-1.760475));
#46867=CARTESIAN_POINT('Ctrl Pts',(0.616798119179157,-0.599398222050533,
-1.760475));
#46868=CARTESIAN_POINT('Ctrl Pts',(0.587194500700165,-0.624245366063714,
-1.760475));
#46869=CARTESIAN_POINT('Ctrl Pts',(0.555989358652953,-0.647004098426802,
-1.760475));
#46870=CARTESIAN_POINT('Ctrl Pts',(0.535293767266585,-0.662097938562045,
-1.760475));
#46871=CARTESIAN_POINT('Ctrl Pts',(0.513893228447004,-0.676272337278064,
-1.760475));
#46872=CARTESIAN_POINT('Ctrl Pts',(0.491830465822602,-0.689450798018773,
-1.760475));
#46873=CARTESIAN_POINT('Origin',(0.,0.,-1.760475));
#46874=CARTESIAN_POINT('Origin',(0.,0.,-2.22262968985462));
#46875=CARTESIAN_POINT('Ctrl Pts',(0.491830465822599,-0.689450798018774,
-1.760475));
#46876=CARTESIAN_POINT('Ctrl Pts',(0.605635182346436,-0.608266430836124,
-1.75390724228836));
#46877=CARTESIAN_POINT('Ctrl Pts',(0.79216447554976,-0.388547169429118,
-1.74077172686508));
#46878=CARTESIAN_POINT('Ctrl Pts',(0.88161996364164,0.0346345312550622,
-1.72106845373015));
#46879=CARTESIAN_POINT('Ctrl Pts',(0.759268494074124,0.449392048212061,
-1.70136518059523));
#46880=CARTESIAN_POINT('Ctrl Pts',(0.454502118692952,0.756233452283398,
-1.6816619074603));
#46881=CARTESIAN_POINT('Ctrl Pts',(0.0405418686236695,0.881364469834283,
-1.66195863432538));
#46882=CARTESIAN_POINT('Ctrl Pts',(-0.383158700471979,0.79476040598,-1.64225536119046));
#46883=CARTESIAN_POINT('Ctrl Pts',(-0.714805313372813,0.517208687205868,
-1.62255208805553));
#46884=CARTESIAN_POINT('Ctrl Pts',(-0.835534807601658,0.213858991565929,
-1.60767686427692));
#46885=CARTESIAN_POINT('Ctrl Pts',(-0.846921218466673,0.0370517561408366,
-1.59936939820995));
#46886=CARTESIAN_POINT('Ctrl Pts',(-0.846885554371379,2.10899746275542E-5,
-1.59762968985462));
#46887=CARTESIAN_POINT('Ctrl Pts',(0.574658804691352,-0.805560043581921,
-1.84281958214317));
#46888=CARTESIAN_POINT('Ctrl Pts',(0.707629181498825,-0.710703554106881,
-1.83625182443153));
#46889=CARTESIAN_POINT('Ctrl Pts',(0.925571558234001,-0.453981742625281,
-1.82311630900825));
#46890=CARTESIAN_POINT('Ctrl Pts',(1.03009209413448,0.0404672742238311,
-1.80341303587332));
#46891=CARTESIAN_POINT('Ctrl Pts',(0.887135620024441,0.525073404778649,
-1.7837097627384));
#46892=CARTESIAN_POINT('Ctrl Pts',(0.531044053606855,0.883589451966854,
-1.76400648960347));
#46893=CARTESIAN_POINT('Ctrl Pts',(0.0473694563110631,1.02979357304613,
-1.74430321646855));
#46894=CARTESIAN_POINT('Ctrl Pts',(-0.447685810703192,0.928604664927808,
-1.72459994333363));
#46895=CARTESIAN_POINT('Ctrl Pts',(-0.835184470085288,0.60431092951634,
-1.7048966701987));
#46896=CARTESIAN_POINT('Ctrl Pts',(-1.02203007614907,0.134835279898603,
-1.68519339706378));
#46897=CARTESIAN_POINT('Ctrl Pts',(-0.963332906852676,-0.367036471470568,
-1.66549012392885));
#46898=CARTESIAN_POINT('Ctrl Pts',(-0.673194989019042,-0.780726729017107,
-1.64578685079393));
#46899=CARTESIAN_POINT('Ctrl Pts',(-0.221321950521705,-1.00684785792862,
-1.62608357765901));
#46900=CARTESIAN_POINT('Ctrl Pts',(0.283723690388641,-0.991073512081083,
-1.60638030452408));
#46901=CARTESIAN_POINT('Ctrl Pts',(0.720604707801549,-0.737193851560317,
-1.58667703138916));
#46902=CARTESIAN_POINT('Ctrl Pts',(0.984360422706338,-0.306203283667381,
-1.56697375825423));
#46903=CARTESIAN_POINT('Ctrl Pts',(1.01162351797873,0.198352600005484,-1.54727048511931));
#46904=CARTESIAN_POINT('Ctrl Pts',(0.795844033690379,0.655254281948304,
-1.52756721198439));
#46905=CARTESIAN_POINT('Ctrl Pts',(0.388862997423207,0.954731095583577,
-1.50786393884946));
#46906=CARTESIAN_POINT('Ctrl Pts',(-0.111542385241397,1.0248337400704,-1.48816066571454));
#46907=CARTESIAN_POINT('Ctrl Pts',(-0.585149706610647,0.848720046844145,
-1.46845739257961));
#46908=CARTESIAN_POINT('Ctrl Pts',(-0.918174794088913,0.468701338919505,
-1.44875411944469));
#46909=CARTESIAN_POINT('Ctrl Pts',(-1.03060836078115,-0.0239228797397841,
-1.42905084630976));
#46910=CARTESIAN_POINT('Ctrl Pts',(-0.895438239052798,-0.510799625582625,
-1.40934757317484));
#46911=CARTESIAN_POINT('Ctrl Pts',(-0.545139054546205,-0.874956746772044,
-1.38964430003991));
#46912=CARTESIAN_POINT('Ctrl Pts',(-0.0638701964516418,-1.0289054842277,
-1.36994102690499));
#46913=CARTESIAN_POINT('Ctrl Pts',(0.432743478184231,-0.935659649435702,
-1.35023775377007));
#46914=CARTESIAN_POINT('Ctrl Pts',(0.82539051969619,-0.617621556844013,
-1.33053448063514));
#46915=CARTESIAN_POINT('Ctrl Pts',(1.01973746502858,-0.151199867403416,
-1.31083120750022));
#46916=CARTESIAN_POINT('Ctrl Pts',(0.969092454955847,0.351547594549289,
-1.2911279343653));
#46917=CARTESIAN_POINT('Ctrl Pts',(0.685622954609774,0.769835736762807,
-1.27142466123037));
#46918=CARTESIAN_POINT('Ctrl Pts',(0.237432519630045,1.00317082100098,-1.25172138809545));
#46919=CARTESIAN_POINT('Ctrl Pts',(-0.267801085043643,0.995494086539286,
-1.23201811496052));
#46920=CARTESIAN_POINT('Ctrl Pts',(-0.708695471306245,0.748649869054587,
-1.2123148418256));
#46921=CARTESIAN_POINT('Ctrl Pts',(-0.979325750132951,0.321942498921626,
-1.19261156869068));
#46922=CARTESIAN_POINT('Ctrl Pts',(-1.01467298922463,-0.182111565869176,
-1.17290829555575));
#46923=CARTESIAN_POINT('Ctrl Pts',(-0.806245013369315,-0.642413321703791,
-1.15320502242083));
#46924=CARTESIAN_POINT('Ctrl Pts',(-0.404116649781944,-0.948375258457533,
-1.1335017492859));
#46925=CARTESIAN_POINT('Ctrl Pts',(0.0951007505792697,-1.02649001199458,
-1.11379847615098));
#46926=CARTESIAN_POINT('Ctrl Pts',(0.571470192868989,-0.857990510523082,
-1.09409520301605));
#46927=CARTESIAN_POINT('Ctrl Pts',(0.910543904827996,-0.483358764134844,
-1.07439192988113));
#46928=CARTESIAN_POINT('Ctrl Pts',(1.0308594173717,0.00739993928763064,
-1.05468865674621));
#46929=CARTESIAN_POINT('Ctrl Pts',(0.90351092513889,0.496380807082673,-1.03498538361128));
#46930=CARTESIAN_POINT('Ctrl Pts',(0.559093907064072,0.866106171649417,
-1.01528211047636));
#46931=CARTESIAN_POINT('Ctrl Pts',(0.0803545616803817,1.02774950347959,
-0.995578837341433));
#46932=CARTESIAN_POINT('Ctrl Pts',(-0.417689969466237,0.94247598743558,
-0.97587556420651));
#46933=CARTESIAN_POINT('Ctrl Pts',(-0.815384473393104,0.630772588208167,
-0.956172291071584));
#46934=CARTESIAN_POINT('Ctrl Pts',(-1.01718283405342,0.1675260564582,-0.936469017936662));
#46935=CARTESIAN_POINT('Ctrl Pts',(-0.974602989474174,-0.335968615191032,
-0.916765744801736));
#46936=CARTESIAN_POINT('Ctrl Pts',(-0.697874748544491,-0.758746817343798,
-0.897062471666814));
#46937=CARTESIAN_POINT('Ctrl Pts',(-0.253482079134731,-0.999236074730547,
-0.877359198531888));
#46938=CARTESIAN_POINT('Ctrl Pts',(0.251809667103219,-0.999658836323045,
-0.857655925396965));
#46939=CARTESIAN_POINT('Ctrl Pts',(0.69660413355182,-0.75991353363649,-0.837952652262041));
#46940=CARTESIAN_POINT('Ctrl Pts',(0.974039436809005,-0.337598982560928,
-0.818249379127116));
#46941=CARTESIAN_POINT('Ctrl Pts',(1.01746173725982,0.165823733818778,-0.798546105992192));
#46942=CARTESIAN_POINT('Ctrl Pts',(0.816438825967693,0.629407293362469,
-0.778842832857268));
#46943=CARTESIAN_POINT('Ctrl Pts',(0.419266463172544,0.941775732509693,
-0.759139559722345));
#46944=CARTESIAN_POINT('Ctrl Pts',(-0.0786346795008153,1.02788252473966,
-0.739436286587419));
#46945=CARTESIAN_POINT('Ctrl Pts',(-0.557643838154491,0.867040510733896,
-0.719733013452497));
#46946=CARTESIAN_POINT('Ctrl Pts',(-0.902679048596748,0.497891988999522,
-0.700029740317572));
#46947=CARTESIAN_POINT('Ctrl Pts',(-1.03084559156011,0.00912490253774741,
-0.680326467182647));
#46948=CARTESIAN_POINT('Ctrl Pts',(-0.911351451398881,-0.481834442022157,
-0.660623194047724));
#46949=CARTESIAN_POINT('Ctrl Pts',(-0.572905098734823,-0.857033047979255,
-0.640919920912798));
#46950=CARTESIAN_POINT('Ctrl Pts',(-0.0968182795654776,-1.02632943942368,
-0.621216647777876));
#46951=CARTESIAN_POINT('Ctrl Pts',(0.402529134066059,-0.949050153423805,
-0.60151337464295));
#46952=CARTESIAN_POINT('Ctrl Pts',(0.805168911615982,-0.643761540673181,
-0.581810101508027));
#46953=CARTESIAN_POINT('Ctrl Pts',(1.01436683491972,-0.183809199193264,
-0.562106828373103));
#46954=CARTESIAN_POINT('Ctrl Pts',(0.97986309684008,0.320303307693771,-0.542403555238179));
#46955=CARTESIAN_POINT('Ctrl Pts',(0.70994722149712,0.74746293567104,-0.522700282103255));
#46956=CARTESIAN_POINT('Ctrl Pts',(0.269466505632264,0.995044571763327,
-0.50299700896833));
#46957=CARTESIAN_POINT('Ctrl Pts',(-0.23575354585651,1.00356672080292,-0.483293735833407));
#46958=CARTESIAN_POINT('Ctrl Pts',(-0.68433380140946,0.770981936139643,
-0.463590462698482));
#46959=CARTESIAN_POINT('Ctrl Pts',(-0.968502840906551,0.353168719194655,
-0.443887189563558));
#46960=CARTESIAN_POINT('Ctrl Pts',(-1.01998904594358,-0.149493292983739,
-0.424183916428634));
#46961=CARTESIAN_POINT('Ctrl Pts',(-0.826422851232646,-0.616239536706045,
-0.40448064329371));
#46962=CARTESIAN_POINT('Ctrl Pts',(-0.434308546660483,-0.934934214942325,
-0.384777370158786));
#46963=CARTESIAN_POINT('Ctrl Pts',(0.0621484066991229,-1.02901091908753,
-0.365074097023862));
#46964=CARTESIAN_POINT('Ctrl Pts',(0.54367418788479,-0.875867724115407,
-0.345370823888937));
#46965=CARTESIAN_POINT('Ctrl Pts',(0.894582260757255,-0.512297275439298,
-0.325667550754014));
#46966=CARTESIAN_POINT('Ctrl Pts',(1.03056685826814,-0.0256474068051044,
-0.305964277619089));
#46967=CARTESIAN_POINT('Ctrl Pts',(0.918957859857471,0.467164282243796,
-0.286261004484165));
#46968=CARTESIAN_POINT('Ctrl Pts',(0.586568968558927,0.847739679244646,
-0.266557731349241));
#46969=CARTESIAN_POINT('Ctrl Pts',(0.113257341734262,1.02464571211618,-0.246854458214317));
#46970=CARTESIAN_POINT('Ctrl Pts',(-0.387265307077567,0.955380348967222,
-0.227151185079393));
#46971=CARTESIAN_POINT('Ctrl Pts',(-0.794745589415275,0.656585292791054,
-0.207447911944469));
#46972=CARTESIAN_POINT('Ctrl Pts',(-1.01129191299364,0.200044683869197,
-0.187744638809545));
#46973=CARTESIAN_POINT('Ctrl Pts',(-0.984868017254482,-0.304554850671511,
-0.168041365674621));
#46974=CARTESIAN_POINT('Ctrl Pts',(-0.721844019653508,-0.7359886668888,
-0.148338092539697));
#46975=CARTESIAN_POINT('Ctrl Pts',(-0.285368307933075,-0.990594073043749,
-0.128634819404772));
#46976=CARTESIAN_POINT('Ctrl Pts',(0.219610032591509,-1.00722329017286,
-0.108931546269848));
#46977=CARTESIAN_POINT('Ctrl Pts',(0.671944475147084,-0.78183934050936,
-0.0892282731349243));
#46978=CARTESIAN_POINT('Ctrl Pts',(0.865681796314515,-0.506392760472071,
-0.0760927577116414));
#46979=CARTESIAN_POINT('Ctrl Pts',(0.924091453827287,-0.353856906938908,
-0.0695250000000001));
#46980=CARTESIAN_POINT('Ctrl Pts',(0.547049358401768,-0.766856961727539,
-1.81537138809545));
#46981=CARTESIAN_POINT('Ctrl Pts',(0.673631181781362,-0.676557846349963,
-1.80880363038381));
#46982=CARTESIAN_POINT('Ctrl Pts',(0.881102530672586,-0.43217021822656,
-1.79566811496052));
#46983=CARTESIAN_POINT('Ctrl Pts',(0.980601383970203,0.038523026567575,
-1.7759648418256));
#46984=CARTESIAN_POINT('Ctrl Pts',(0.844513244707669,0.49984628592312,-1.75626156869068));
#46985=CARTESIAN_POINT('Ctrl Pts',(0.505530075302221,0.841137452072369,
-1.73655829555575));
#46986=CARTESIAN_POINT('Ctrl Pts',(0.0450935937485983,0.980317205308848,
-1.71685502242083));
#46987=CARTESIAN_POINT('Ctrl Pts',(-0.426176773959454,0.883989911945206,
-1.6971517492859));
#46988=CARTESIAN_POINT('Ctrl Pts',(-0.795058084514463,0.575276848746182,
-1.67744847615098));
#46989=CARTESIAN_POINT('Ctrl Pts',(-0.972926705134103,0.12835712731848,
-1.65774520301605));
#46990=CARTESIAN_POINT('Ctrl Pts',(-0.917049637661276,-0.349402227180467,
-1.63804192988113));
#46991=CARTESIAN_POINT('Ctrl Pts',(-0.640851377923199,-0.743216762206073,
-1.61833865674621));
#46992=CARTESIAN_POINT('Ctrl Pts',(-0.21068855126679,-0.958473915637432,
-1.59863538361128));
#46993=CARTESIAN_POINT('Ctrl Pts',(0.270092203449057,-0.943457447248438,
-1.57893211047636));
#46994=CARTESIAN_POINT('Ctrl Pts',(0.685983299735323,-0.701775419120918,
-1.55922883734143));
#46995=CARTESIAN_POINT('Ctrl Pts',(0.93706688783237,-0.291491766076259,
-1.53952556420651));
#46996=CARTESIAN_POINT('Ctrl Pts',(0.963020129399458,0.188822761757913,
-1.51982229107159));
#46997=CARTESIAN_POINT('Ctrl Pts',(0.757607756922875,0.623772631000333,
-1.50011901793666));
#46998=CARTESIAN_POINT('Ctrl Pts',(0.370180099060361,0.908861099876003,
-1.48041574480174));
#46999=CARTESIAN_POINT('Ctrl Pts',(-0.106183338326614,0.975595667197877,
-1.46071247166681));
#47000=CARTESIAN_POINT('Ctrl Pts',(-0.557036225595229,0.807943345335459,
-1.44100919853189));
#47001=CARTESIAN_POINT('Ctrl Pts',(-0.874061143597708,0.446182612438484,
-1.42130592539696));
#47002=CARTESIAN_POINT('Ctrl Pts',(-0.981092846618151,-0.0227735064805993,
-1.40160265226204));
#47003=CARTESIAN_POINT('Ctrl Pts',(-0.85241696492467,-0.486258289554828,
-1.38189937912712));
#47004=CARTESIAN_POINT('Ctrl Pts',(-0.518947882803987,-0.832919504658114,
-1.36219610599219));
#47005=CARTESIAN_POINT('Ctrl Pts',(-0.0608015568623043,-0.979471784662089,
-1.34249283285727));
#47006=CARTESIAN_POINT('Ctrl Pts',(0.411952344870764,-0.89070594016416,
-1.32278955972234));
#47007=CARTESIAN_POINT('Ctrl Pts',(0.785734683858569,-0.587947967817332,
-1.30308628658742));
#47008=CARTESIAN_POINT('Ctrl Pts',(0.970744242371342,-0.14393547924128,
-1.2833830134525));
#47009=CARTESIAN_POINT('Ctrl Pts',(0.922532468636458,0.334657512381047,
-1.26367974031757));
#47010=CARTESIAN_POINT('Ctrl Pts',(0.652682242685291,0.7328490269927,-1.24397646718265));
#47011=CARTESIAN_POINT('Ctrl Pts',(0.22602508909107,0.954973541718743,-1.22427319404772));
#47012=CARTESIAN_POINT('Ctrl Pts',(-0.254934598680877,0.94766563548359,
-1.2045699209128));
#47013=CARTESIAN_POINT('Ctrl Pts',(-0.67464624176175,0.712681032971984,
-1.18486664777788));
#47014=CARTESIAN_POINT('Ctrl Pts',(-0.932274105787528,0.306474791719114,
-1.16516337464295));
#47015=CARTESIAN_POINT('Ctrl Pts',(-0.965923088990291,-0.173362027089766,
-1.14546010150803));
#47016=CARTESIAN_POINT('Ctrl Pts',(-0.767509022184385,-0.611548613886739,
-1.1257568283731));
#47017=CARTESIAN_POINT('Ctrl Pts',(-0.384700890646618,-0.902810628546715,
-1.10605355523818));
#47018=CARTESIAN_POINT('Ctrl Pts',(0.090531640972349,-0.977172363641172,
-1.08635028210325));
#47019=CARTESIAN_POINT('Ctrl Pts',(0.544013943234757,-0.816768410167404,
-1.06664700896833));
#47020=CARTESIAN_POINT('Ctrl Pts',(0.86679687993353,-0.460135822577115,
-1.04694373583341));
#47021=CARTESIAN_POINT('Ctrl Pts',(0.981331841210531,0.00704440966789899,
-1.02724046269848));
#47022=CARTESIAN_POINT('Ctrl Pts',(0.860101799313222,0.472532222286882,
-1.00753718956356));
#47023=CARTESIAN_POINT('Ctrl Pts',(0.532232275306405,0.824494154863082,
-0.987833916428634));
#47024=CARTESIAN_POINT('Ctrl Pts',(0.0764939317957849,0.978371342936638,
-0.968130643293711));
#47025=CARTESIAN_POINT('Ctrl Pts',(-0.397622081036563,0.897194787631635,
-0.948427370158785));
#47026=CARTESIAN_POINT('Ctrl Pts',(-0.776209377423594,0.600467158703036,
-0.928724097023862));
#47027=CARTESIAN_POINT('Ctrl Pts',(-0.968312348481428,0.159477277565179,
-0.909020823888938));
#47028=CARTESIAN_POINT('Ctrl Pts',(-0.927778249868891,-0.319827024110592,
-0.889317550754013));
#47029=CARTESIAN_POINT('Ctrl Pts',(-0.664345399947551,-0.722292874012854,
-0.86961427761909));
#47030=CARTESIAN_POINT('Ctrl Pts',(-0.241303548514284,-0.951227840086503,
-0.849911004484165));
#47031=CARTESIAN_POINT('Ctrl Pts',(0.239711487414111,-0.951630290124759,
-0.830207731349241));
#47032=CARTESIAN_POINT('Ctrl Pts',(0.663135831572647,-0.723403535494316,
-0.810504458214317));
#47033=CARTESIAN_POINT('Ctrl Pts',(0.927241773056233,-0.321379060582283,
-0.790801185079393));
#47034=CARTESIAN_POINT('Ctrl Pts',(0.968577851800747,0.157856742910379,
-0.771097911944469));
#47035=CARTESIAN_POINT('Ctrl Pts',(0.777213073694752,0.599167459362714,
-0.751394638809544));
#47036=CARTESIAN_POINT('Ctrl Pts',(0.39912283220146,0.896528176409816,-0.73169136567462));
#47037=CARTESIAN_POINT('Ctrl Pts',(-0.0748566812478484,0.978497973198602,
-0.711988092539697));
#47038=CARTESIAN_POINT('Ctrl Pts',(-0.530851874866792,0.825383603684749,
-0.692284819404772));
#47039=CARTESIAN_POINT('Ctrl Pts',(-0.85930989022746,0.473970799563156,
-0.672581546269849));
#47040=CARTESIAN_POINT('Ctrl Pts',(-0.981318679659197,0.00868649716666914,
-0.652878273134924));
#47041=CARTESIAN_POINT('Ctrl Pts',(-0.867565627979979,-0.458684736424889,
-0.633175000000001));
#47042=CARTESIAN_POINT('Ctrl Pts',(-0.545379909138111,-0.815856948851546,
-0.613471726865076));
#47043=CARTESIAN_POINT('Ctrl Pts',(-0.0921666513859544,-0.977019505769383,
-0.593768453730152));
#47044=CARTESIAN_POINT('Ctrl Pts',(0.383189647023903,-0.90345309822659,
-0.574065180595227));
#47045=CARTESIAN_POINT('Ctrl Pts',(0.766484621672412,-0.612832057760162,
-0.554361907460304));
#47046=CARTESIAN_POINT('Ctrl Pts',(0.965631643849792,-0.174978097727091,
-0.534658634325379));
#47047=CARTESIAN_POINT('Ctrl Pts',(0.932785635705759,0.304914355331165,
-0.514955361190455));
#47048=CARTESIAN_POINT('Ctrl Pts',(0.67583785169308,0.711551125728532,-0.495252088055531));
#47049=CARTESIAN_POINT('Ctrl Pts',(0.256520004241595,0.947237717616896,
-0.475548814920607));
#47050=CARTESIAN_POINT('Ctrl Pts',(-0.224426781507358,0.955350420539488,
-0.455845541785683));
#47051=CARTESIAN_POINT('Ctrl Pts',(-0.651455026769769,0.733940157292244,
-0.436142268650759));
#47052=CARTESIAN_POINT('Ctrl Pts',(-0.921971182557243,0.336200750194329,
-0.416438995515835));
#47053=CARTESIAN_POINT('Ctrl Pts',(-0.970983736097037,-0.142310897082741,
-0.396735722380911));
#47054=CARTESIAN_POINT('Ctrl Pts',(-0.786717417090993,-0.586632346750361,
-0.377032449245986));
#47055=CARTESIAN_POINT('Ctrl Pts',(-0.413442219730069,-0.890015359125594,
-0.357329176111063));
#47056=CARTESIAN_POINT('Ctrl Pts',(0.0591624903906386,-0.979572153910683,
-0.337625902976138));
#47057=CARTESIAN_POINT('Ctrl Pts',(0.5175533955696,-0.833786714152053,-0.317922629841214));
#47058=CARTESIAN_POINT('Ctrl Pts',(0.851602112052742,-0.48768398491791,
-0.29821935670629));
#47059=CARTESIAN_POINT('Ctrl Pts',(0.98105333809078,-0.0244151787510444,
-0.278516083571366));
#47060=CARTESIAN_POINT('Ctrl Pts',(0.874806587020447,0.444719403554519,
-0.258812810436442));
#47061=CARTESIAN_POINT('Ctrl Pts',(0.558387299192069,0.807010079435893,
-0.239109537301518));
#47062=CARTESIAN_POINT('Ctrl Pts',(0.107815899842159,0.975416673034951,
-0.219406264166593));
#47063=CARTESIAN_POINT('Ctrl Pts',(-0.36865916964734,0.909479159921484,
-0.19970299103167));
#47064=CARTESIAN_POINT('Ctrl Pts',(-0.756562087334191,0.625039693510482,
-0.179999717896746));
#47065=CARTESIAN_POINT('Ctrl Pts',(-0.962704456355113,0.190433549558341,
-0.160296444761821));
#47066=CARTESIAN_POINT('Ctrl Pts',(-0.93755009503223,-0.289922531940463,
-0.140593171626897));
#47067=CARTESIAN_POINT('Ctrl Pts',(-0.687163068926953,-0.700628137471483,
-0.120889898491973));
#47068=CARTESIAN_POINT('Ctrl Pts',(-0.271657805446542,-0.943001042829635,
-0.101186625357049));
#47069=CARTESIAN_POINT('Ctrl Pts',(0.209058882326361,-0.958831310262997,
-0.0814833522221245));
#47070=CARTESIAN_POINT('Ctrl Pts',(0.63966094491192,-0.744275918348846,
-0.0617800790872008));
#47071=CARTESIAN_POINT('Ctrl Pts',(0.824090168614572,-0.482063152002576,
-0.0486445636639179));
#47072=CARTESIAN_POINT('Ctrl Pts',(0.879693537789418,-0.336855874001501,
-0.0420768059522765));
#47073=CARTESIAN_POINT('Ctrl Pts',(0.519439912112184,-0.728153879873157,
-1.78792319404772));
#47074=CARTESIAN_POINT('Ctrl Pts',(0.639633182063899,-0.642412138593043,
-1.78135543633608));
#47075=CARTESIAN_POINT('Ctrl Pts',(0.836633503111173,-0.410358693827839,
-1.7682199209128));
#47076=CARTESIAN_POINT('Ctrl Pts',(0.931110673805921,0.0365787789113189,
-1.74851664777787));
#47077=CARTESIAN_POINT('Ctrl Pts',(0.801890869390896,0.47461916706759,-1.72881337464295));
#47078=CARTESIAN_POINT('Ctrl Pts',(0.480016096997586,0.798685452177885,
-1.70911010150802));
#47079=CARTESIAN_POINT('Ctrl Pts',(0.0428177311861338,0.930840837571564,
-1.68940682837311));
#47080=CARTESIAN_POINT('Ctrl Pts',(-0.404667737215717,0.839375158962604,
-1.66970355523818));
#47081=CARTESIAN_POINT('Ctrl Pts',(-0.754931698943638,0.546242767976024,
-1.65000028210326));
#47082=CARTESIAN_POINT('Ctrl Pts',(-0.923823334119134,0.121878974738357,
-1.63029700896833));
#47083=CARTESIAN_POINT('Ctrl Pts',(-0.870766368469874,-0.331767982890366,
-1.61059373583341));
#47084=CARTESIAN_POINT('Ctrl Pts',(-0.608507766827356,-0.705706795395039,
-1.59089046269848));
#47085=CARTESIAN_POINT('Ctrl Pts',(-0.200055152011874,-0.910099973346243,
-1.57118718956356));
#47086=CARTESIAN_POINT('Ctrl Pts',(0.256460716509473,-0.895841382415795,
-1.55148391642863));
#47087=CARTESIAN_POINT('Ctrl Pts',(0.651361891669097,-0.666356986681518,
-1.53178064329371));
#47088=CARTESIAN_POINT('Ctrl Pts',(0.889773352958402,-0.276780248485138,
-1.51207737015879));
#47089=CARTESIAN_POINT('Ctrl Pts',(0.914416740820184,0.179292923510344,
-1.49237409702386));
#47090=CARTESIAN_POINT('Ctrl Pts',(0.719371480155372,0.592290980052361,
-1.47267082388894));
#47091=CARTESIAN_POINT('Ctrl Pts',(0.351497200697514,0.862991104168431,
-1.45296755075401));
#47092=CARTESIAN_POINT('Ctrl Pts',(-0.100824291411831,0.926357594325357,
-1.43326427761909));
#47093=CARTESIAN_POINT('Ctrl Pts',(-0.528922744579813,0.767166643826773,
-1.41356100448417));
#47094=CARTESIAN_POINT('Ctrl Pts',(-0.829947493106503,0.423663885957463,
-1.39385773134924));
#47095=CARTESIAN_POINT('Ctrl Pts',(-0.931577332455155,-0.0216241332214148,
-1.37415445821432));
#47096=CARTESIAN_POINT('Ctrl Pts',(-0.809395690796543,-0.46171695352703,
-1.35445118507939));
#47097=CARTESIAN_POINT('Ctrl Pts',(-0.492756711061769,-0.790882262544183,
-1.33474791194447));
#47098=CARTESIAN_POINT('Ctrl Pts',(-0.0577329172729664,-0.930038085096481,
-1.31504463880955));
#47099=CARTESIAN_POINT('Ctrl Pts',(0.391161211557297,-0.845752230892618,
-1.29534136567462));
#47100=CARTESIAN_POINT('Ctrl Pts',(0.746078848020947,-0.558274378790652,
-1.2756380925397));
#47101=CARTESIAN_POINT('Ctrl Pts',(0.921751019714107,-0.136671091079143,
-1.25593481940477));
#47102=CARTESIAN_POINT('Ctrl Pts',(0.87597248231707,0.317767430212804,-1.23623154626985));
#47103=CARTESIAN_POINT('Ctrl Pts',(0.619741530760809,0.695862317222595,
-1.21652827313492));
#47104=CARTESIAN_POINT('Ctrl Pts',(0.214617658552094,0.906776262436506,
-1.196825));
#47105=CARTESIAN_POINT('Ctrl Pts',(-0.242068112318111,0.899837184427893,
-1.17712172686508));
#47106=CARTESIAN_POINT('Ctrl Pts',(-0.640597012217254,0.67671219688938,
-1.15741845373015));
#47107=CARTESIAN_POINT('Ctrl Pts',(-0.885222461442106,0.291007084516601,
-1.13771518059523));
#47108=CARTESIAN_POINT('Ctrl Pts',(-0.917173188755948,-0.164612488310355,
-1.1180119074603));
#47109=CARTESIAN_POINT('Ctrl Pts',(-0.728773030999457,-0.58068390606969,
-1.09830863432538));
#47110=CARTESIAN_POINT('Ctrl Pts',(-0.36528513151129,-0.857245998635898,
-1.07860536119046));
#47111=CARTESIAN_POINT('Ctrl Pts',(0.0859625313654273,-0.927854715287762,
-1.05890208805553));
#47112=CARTESIAN_POINT('Ctrl Pts',(0.516557693600527,-0.775546309811726,
-1.03919881492061));
#47113=CARTESIAN_POINT('Ctrl Pts',(0.823049855039062,-0.436912881019387,
-1.01949554178568));
#47114=CARTESIAN_POINT('Ctrl Pts',(0.931804265049363,0.00668888004816687,
-0.999792268650759));
#47115=CARTESIAN_POINT('Ctrl Pts',(0.816692673487552,0.448683637491092,
-0.980088995515835));
#47116=CARTESIAN_POINT('Ctrl Pts',(0.505370643548739,0.782882138076745,
-0.96038572238091));
#47117=CARTESIAN_POINT('Ctrl Pts',(0.0726333019111879,0.928993182393693,
-0.940682449245987));
#47118=CARTESIAN_POINT('Ctrl Pts',(-0.377554192606889,0.851913587827687,
-0.920979176111061));
#47119=CARTESIAN_POINT('Ctrl Pts',(-0.737034281454082,0.570161729197906,
-0.901275902976139));
#47120=CARTESIAN_POINT('Ctrl Pts',(-0.919441862909439,0.151428498672156,
-0.881572629841214));
#47121=CARTESIAN_POINT('Ctrl Pts',(-0.880953510263607,-0.303685433030151,
-0.86186935670629));
#47122=CARTESIAN_POINT('Ctrl Pts',(-0.630816051350612,-0.68583893068191,
-0.842166083571366));
#47123=CARTESIAN_POINT('Ctrl Pts',(-0.229125017893837,-0.903219605442459,
-0.822462810436442));
#47124=CARTESIAN_POINT('Ctrl Pts',(0.227613307725003,-0.903601743926474,
-0.802759537301517));
#47125=CARTESIAN_POINT('Ctrl Pts',(0.629667529593472,-0.686893537352141,
-0.783056264166594));
#47126=CARTESIAN_POINT('Ctrl Pts',(0.880444109303463,-0.305159138603638,
-0.763352991031669));
#47127=CARTESIAN_POINT('Ctrl Pts',(0.919693966341668,0.14988975200198,-0.743649717896745));
#47128=CARTESIAN_POINT('Ctrl Pts',(0.737987321421813,0.56892762536296,-0.723946444761821));
#47129=CARTESIAN_POINT('Ctrl Pts',(0.378979201230375,0.851280620309938,
-0.704243171626897));
#47130=CARTESIAN_POINT('Ctrl Pts',(-0.0710786829948813,0.929113421657545,
-0.684539898491973));
#47131=CARTESIAN_POINT('Ctrl Pts',(-0.504059911579092,0.783726696635601,
-0.664836625357049));
#47132=CARTESIAN_POINT('Ctrl Pts',(-0.815940731858172,0.450049610126791,
-0.645133352222125));
#47133=CARTESIAN_POINT('Ctrl Pts',(-0.931791767758281,0.00824809179559103,
-0.6254300790872));
#47134=CARTESIAN_POINT('Ctrl Pts',(-0.823779804561077,-0.435535030827622,
-0.605726805952277));
#47135=CARTESIAN_POINT('Ctrl Pts',(-0.5178547195414,-0.774680849723837,
-0.586023532817352));
#47136=CARTESIAN_POINT('Ctrl Pts',(-0.0875150232064309,-0.927709572115086,
-0.566320259682429));
#47137=CARTESIAN_POINT('Ctrl Pts',(0.363850159981747,-0.857856043029375,
-0.546616986547504));
#47138=CARTESIAN_POINT('Ctrl Pts',(0.727800331728844,-0.581902574847143,
-0.52691371341258));
#47139=CARTESIAN_POINT('Ctrl Pts',(0.91689645277986,-0.16614699626092,-0.507210440277656));
#47140=CARTESIAN_POINT('Ctrl Pts',(0.885708174571438,0.28952540296856,-0.487507167142732));
#47141=CARTESIAN_POINT('Ctrl Pts',(0.64172848188904,0.675639315786023,-0.467803894007807));
#47142=CARTESIAN_POINT('Ctrl Pts',(0.243573502850927,0.899430863470464,
-0.448100620872884));
#47143=CARTESIAN_POINT('Ctrl Pts',(-0.213100017158207,0.907134120276057,
-0.428397347737959));
#47144=CARTESIAN_POINT('Ctrl Pts',(-0.618576252130077,0.696898378444844,
-0.408694074603035));
#47145=CARTESIAN_POINT('Ctrl Pts',(-0.875439524207936,0.319232781194004,
-0.388990801468111));
#47146=CARTESIAN_POINT('Ctrl Pts',(-0.921978426250493,-0.135128501181744,
-0.369287528333187));
#47147=CARTESIAN_POINT('Ctrl Pts',(-0.74701198294934,-0.557025156794675,
-0.349584255198263));
#47148=CARTESIAN_POINT('Ctrl Pts',(-0.392575892799654,-0.845096503308866,
-0.329880982063339));
#47149=CARTESIAN_POINT('Ctrl Pts',(0.0561765740821534,-0.930133388733834,
-0.310177708928415));
#47150=CARTESIAN_POINT('Ctrl Pts',(0.49143260325441,-0.791705704188701,
-0.29047443579349));
#47151=CARTESIAN_POINT('Ctrl Pts',(0.808621963348227,-0.46307069439652,
-0.270771162658566));
#47152=CARTESIAN_POINT('Ctrl Pts',(0.931539817913425,-0.0231829506969853,
-0.251067889523642));
#47153=CARTESIAN_POINT('Ctrl Pts',(0.830655314183421,0.422274524865243,
-0.231364616388718));
#47154=CARTESIAN_POINT('Ctrl Pts',(0.530205629825212,0.766280479627141,
-0.211661343253794));
#47155=CARTESIAN_POINT('Ctrl Pts',(0.102374457950055,0.926187633953719,
-0.19195807011887));
#47156=CARTESIAN_POINT('Ctrl Pts',(-0.350053032217113,0.863577970875746,
-0.172254796983946));
#47157=CARTESIAN_POINT('Ctrl Pts',(-0.718378585253108,0.593494094229909,
-0.152551523849022));
#47158=CARTESIAN_POINT('Ctrl Pts',(-0.914116999716585,0.180822415247486,
-0.132848250714098));
#47159=CARTESIAN_POINT('Ctrl Pts',(-0.890232172809978,-0.275290213209414,
-0.113144977579174));
#47160=CARTESIAN_POINT('Ctrl Pts',(-0.652482118200398,-0.665267608054165,
-0.0934417044442497));
#47161=CARTESIAN_POINT('Ctrl Pts',(-0.25794730296001,-0.895408012615521,
-0.0737384313093254));
#47162=CARTESIAN_POINT('Ctrl Pts',(0.198507732061213,-0.91043933035314,
-0.054035158174401));
#47163=CARTESIAN_POINT('Ctrl Pts',(0.607377414676756,-0.706712496188332,
-0.0343318850394772));
#47164=CARTESIAN_POINT('Ctrl Pts',(0.78249854091463,-0.457733543533081,
-0.0211963696161944));
#47165=CARTESIAN_POINT('Ctrl Pts',(0.835295621751549,-0.319854841064094,
-0.014628611904553));
#47166=CARTESIAN_POINT('Ctrl Pts',(0.491830465822599,-0.689450798018774,
-1.760475));
#47167=CARTESIAN_POINT('Ctrl Pts',(0.605635182346436,-0.608266430836124,
-1.75390724228836));
#47168=CARTESIAN_POINT('Ctrl Pts',(0.79216447554976,-0.388547169429118,
-1.74077172686508));
#47169=CARTESIAN_POINT('Ctrl Pts',(0.88161996364164,0.0346345312550622,
-1.72106845373015));
#47170=CARTESIAN_POINT('Ctrl Pts',(0.759268494074124,0.449392048212061,
-1.70136518059523));
#47171=CARTESIAN_POINT('Ctrl Pts',(0.454502118692952,0.756233452283398,
-1.6816619074603));
#47172=CARTESIAN_POINT('Ctrl Pts',(0.0405418686236695,0.881364469834283,
-1.66195863432538));
#47173=CARTESIAN_POINT('Ctrl Pts',(-0.383158700471979,0.79476040598,-1.64225536119046));
#47174=CARTESIAN_POINT('Ctrl Pts',(-0.714805313372813,0.517208687205868,
-1.62255208805553));
#47175=CARTESIAN_POINT('Ctrl Pts',(-0.874719963104165,0.115400822158233,
-1.60284881492061));
#47176=CARTESIAN_POINT('Ctrl Pts',(-0.824483099278473,-0.314133738600265,
-1.58314554178568));
#47177=CARTESIAN_POINT('Ctrl Pts',(-0.576164155731512,-0.668196828584006,
-1.56344226865076));
#47178=CARTESIAN_POINT('Ctrl Pts',(-0.189421752756959,-0.861726031055052,
-1.54373899551583));
#47179=CARTESIAN_POINT('Ctrl Pts',(0.242829229569888,-0.848225317583151,
-1.52403572238091));
#47180=CARTESIAN_POINT('Ctrl Pts',(0.616740483602872,-0.630938554242118,
-1.50433244924599));
#47181=CARTESIAN_POINT('Ctrl Pts',(0.842479818084434,-0.262068730894017,
-1.48462917611106));
#47182=CARTESIAN_POINT('Ctrl Pts',(0.865813352240911,0.169763085262774,
-1.46492590297614));
#47183=CARTESIAN_POINT('Ctrl Pts',(0.681135203387868,0.560809329104389,
-1.44522262984121));
#47184=CARTESIAN_POINT('Ctrl Pts',(0.332814302334667,0.81712110846086,-1.42551935670629));
#47185=CARTESIAN_POINT('Ctrl Pts',(-0.0954652444970479,0.877119521452837,
-1.40581608357137));
#47186=CARTESIAN_POINT('Ctrl Pts',(-0.500809263564396,0.726389942318086,
-1.38611281043644));
#47187=CARTESIAN_POINT('Ctrl Pts',(-0.785833842615297,0.401145159476442,
-1.36640953730152));
#47188=CARTESIAN_POINT('Ctrl Pts',(-0.882061818292162,-0.0204747599622306,
-1.34670626416659));
#47189=CARTESIAN_POINT('Ctrl Pts',(-0.766374416668415,-0.437175617499231,
-1.32700299103167));
#47190=CARTESIAN_POINT('Ctrl Pts',(-0.466565539319551,-0.748845020430254,
-1.30729971789674));
#47191=CARTESIAN_POINT('Ctrl Pts',(-0.0546642776836284,-0.880604385530872,
-1.28759644476182));
#47192=CARTESIAN_POINT('Ctrl Pts',(0.37037007824383,-0.800798521621077,
-1.2678931716269));
#47193=CARTESIAN_POINT('Ctrl Pts',(0.706423012183327,-0.52860078976397,
-1.24818989849197));
#47194=CARTESIAN_POINT('Ctrl Pts',(0.872757797056872,-0.129406702917007,
-1.22848662535705));
#47195=CARTESIAN_POINT('Ctrl Pts',(0.829412495997682,0.300877348044562,
-1.20878335222212));
#47196=CARTESIAN_POINT('Ctrl Pts',(0.586800818836326,0.658875607452487,
-1.1890800790872));
#47197=CARTESIAN_POINT('Ctrl Pts',(0.20321022801312,0.858578983154271,-1.16937680595228));
#47198=CARTESIAN_POINT('Ctrl Pts',(-0.229201625955346,0.852008733372195,
-1.14967353281735));
#47199=CARTESIAN_POINT('Ctrl Pts',(-0.606547782672759,0.640743360806779,
-1.12997025968243));
#47200=CARTESIAN_POINT('Ctrl Pts',(-0.838170817096684,0.275539377314088,
-1.11026698654751));
#47201=CARTESIAN_POINT('Ctrl Pts',(-0.868423288521605,-0.155862949530944,
-1.09056371341258));
#47202=CARTESIAN_POINT('Ctrl Pts',(-0.690037039814528,-0.549819198252638,
-1.07086044027766));
#47203=CARTESIAN_POINT('Ctrl Pts',(-0.345869372375964,-0.811681368725081,
-1.05115716714273));
#47204=CARTESIAN_POINT('Ctrl Pts',(0.0813934217585064,-0.878537066934349,
-1.03145389400781));
#47205=CARTESIAN_POINT('Ctrl Pts',(0.489101443966296,-0.734324209456049,
-1.01175062087288));
#47206=CARTESIAN_POINT('Ctrl Pts',(0.779302830144596,-0.413689939461657,
-0.99204734773796));
#47207=CARTESIAN_POINT('Ctrl Pts',(0.882276688888196,0.00633335042843485,
-0.972344074603035));
#47208=CARTESIAN_POINT('Ctrl Pts',(0.773283547661882,0.424835052695301,
-0.952640801468111));
#47209=CARTESIAN_POINT('Ctrl Pts',(0.478509011791072,0.74127012129041,-0.932937528333187));
#47210=CARTESIAN_POINT('Ctrl Pts',(0.0687726720265907,0.879615021850747,
-0.913234255198264));
#47211=CARTESIAN_POINT('Ctrl Pts',(-0.357486304177214,0.806632388023741,
-0.893530982063338));
#47212=CARTESIAN_POINT('Ctrl Pts',(-0.697859185484572,0.539856299692775,
-0.873827708928416));
#47213=CARTESIAN_POINT('Ctrl Pts',(-0.870571377337449,0.143379719779135,
-0.85412443579349));
#47214=CARTESIAN_POINT('Ctrl Pts',(-0.834128770658324,-0.287543841949712,
-0.834421162658567));
#47215=CARTESIAN_POINT('Ctrl Pts',(-0.597286702753671,-0.649384987350965,
-0.814717889523642));
#47216=CARTESIAN_POINT('Ctrl Pts',(-0.21694648727339,-0.855211370798415,
-0.795014616388718));
#47217=CARTESIAN_POINT('Ctrl Pts',(0.215515128035896,-0.855573197728189,
-0.775311343253795));
#47218=CARTESIAN_POINT('Ctrl Pts',(0.596199227614297,-0.650383539209966,
-0.75560807011887));
#47219=CARTESIAN_POINT('Ctrl Pts',(0.833646445550691,-0.288939216624994,
-0.735904796983946));
#47220=CARTESIAN_POINT('Ctrl Pts',(0.870810080882589,0.141922761093581,
-0.716201523849022));
#47221=CARTESIAN_POINT('Ctrl Pts',(0.698761569148873,0.538687791363206,
-0.696498250714097));
#47222=CARTESIAN_POINT('Ctrl Pts',(0.358835570259291,0.806033064210061,
-0.676794977579174));
#47223=CARTESIAN_POINT('Ctrl Pts',(-0.0673006847419141,0.879728870116488,
-0.657091704444249));
#47224=CARTESIAN_POINT('Ctrl Pts',(-0.477267948291393,0.742069789586453,
-0.637388431309326));
#47225=CARTESIAN_POINT('Ctrl Pts',(-0.772571573488883,0.426128420690425,
-0.617685158174401));
#47226=CARTESIAN_POINT('Ctrl Pts',(-0.882264855857366,0.00780968642451235,
-0.597981885039478));
#47227=CARTESIAN_POINT('Ctrl Pts',(-0.779993981142175,-0.412385325230355,
-0.578278611904553));
#47228=CARTESIAN_POINT('Ctrl Pts',(-0.490329529944689,-0.733504750596127,
-0.558575338769629));
#47229=CARTESIAN_POINT('Ctrl Pts',(-0.0828633950269074,-0.878399638460791,
-0.538872065634705));
#47230=CARTESIAN_POINT('Ctrl Pts',(0.344510672939591,-0.812258987832161,
-0.51916879249978));
#47231=CARTESIAN_POINT('Ctrl Pts',(0.689116041785277,-0.550973091934125,
-0.499465519364857));
#47232=CARTESIAN_POINT('Ctrl Pts',(0.868161261709926,-0.157315894794747,
-0.479762246229933));
#47233=CARTESIAN_POINT('Ctrl Pts',(0.838630713437117,0.274136450605954,
-0.460058973095008));
#47234=CARTESIAN_POINT('Ctrl Pts',(0.607619112085,0.639727505843516,-0.440355699960084));
#47235=CARTESIAN_POINT('Ctrl Pts',(0.230627001460258,0.851624009324031,
-0.42065242682516));
#47236=CARTESIAN_POINT('Ctrl Pts',(-0.201773252809055,0.858917820012625,
-0.400949153690236));
#47237=CARTESIAN_POINT('Ctrl Pts',(-0.585697477490385,0.659856599597445,
-0.381245880555312));
#47238=CARTESIAN_POINT('Ctrl Pts',(-0.828907865858628,0.302264812193679,
-0.361542607420387));
#47239=CARTESIAN_POINT('Ctrl Pts',(-0.872973116403949,-0.127946105280747,
-0.341839334285464));
#47240=CARTESIAN_POINT('Ctrl Pts',(-0.707306548807687,-0.52741796683899,
-0.322136061150539));
#47241=CARTESIAN_POINT('Ctrl Pts',(-0.37170956586924,-0.800177647492136,
-0.302432788015616));
#47242=CARTESIAN_POINT('Ctrl Pts',(0.053190657773669,-0.880694623556987,
-0.282729514880691));
#47243=CARTESIAN_POINT('Ctrl Pts',(0.46531181093922,-0.749624694225347,
-0.263026241745767));
#47244=CARTESIAN_POINT('Ctrl Pts',(0.765641814643713,-0.438457403875131,
-0.243322968610843));
#47245=CARTESIAN_POINT('Ctrl Pts',(0.88202629773607,-0.0219507226429252,
-0.223619695475919));
#47246=CARTESIAN_POINT('Ctrl Pts',(0.786504041346395,0.399829646175967,
-0.203916422340995));
#47247=CARTESIAN_POINT('Ctrl Pts',(0.502023960458353,0.725550879818389,
-0.184213149206071));
#47248=CARTESIAN_POINT('Ctrl Pts',(0.0969330160579518,0.876958594872486,
-0.164509876071146));
#47249=CARTESIAN_POINT('Ctrl Pts',(-0.331446894786887,0.817676781830008,
-0.144806602936223));
#47250=CARTESIAN_POINT('Ctrl Pts',(-0.680195083172024,0.561948494949336,
-0.125103329801299));
#47251=CARTESIAN_POINT('Ctrl Pts',(-0.865529543078058,0.171211280936631,
-0.105400056666374));
#47252=CARTESIAN_POINT('Ctrl Pts',(-0.842914250587726,-0.260657894478366,
-0.08569678353145));
#47253=CARTESIAN_POINT('Ctrl Pts',(-0.617801167473842,-0.629907078636848,
-0.0659935103965262));
#47254=CARTESIAN_POINT('Ctrl Pts',(-0.244236800473478,-0.847814982401407,
-0.0462902372616019));
#47255=CARTESIAN_POINT('Ctrl Pts',(0.187956581796065,-0.862047350443283,
-0.0265869641266775));
#47256=CARTESIAN_POINT('Ctrl Pts',(0.575093884441593,-0.669149074027817,
-0.00688369099175378));
#47257=CARTESIAN_POINT('Ctrl Pts',(0.740906913214688,-0.433403935063586,
0.0062518244315291));
#47258=CARTESIAN_POINT('Ctrl Pts',(0.790897705713681,-0.302853808126686,
0.0128195821431705));
#47259=CARTESIAN_POINT('Ctrl Pts',(0.924091453827287,-0.353856906938908,
-0.0695250000000001));
#47260=CARTESIAN_POINT('Ctrl Pts',(0.865681796314515,-0.506392760472071,
-0.0760927577116414));
#47261=CARTESIAN_POINT('Ctrl Pts',(0.768813135730799,-0.644116050490716,
-0.0826605154232829));
#47262=CARTESIAN_POINT('Ctrl Pts',(0.644989731679679,-0.750541687110621,
-0.0892282731349242));
#47263=CARTESIAN_POINT('Ctrl Pts',(0.521166327628559,-0.856967323730525,
-0.0957960308465655));
#47264=CARTESIAN_POINT('Ctrl Pts',(0.370388180110033,-0.93209530695169,
-0.102363788558207));
#47265=CARTESIAN_POINT('Ctrl Pts',(0.210836049596674,-0.966887762374088,
-0.108931546269848));
#47266=CARTESIAN_POINT('Ctrl Pts',(0.0512839190833129,-1.00168021779649,
-0.11549930398149));
#47267=CARTESIAN_POINT('Ctrl Pts',(-0.117042194424879,-0.996137145420118,
-0.122067061693131));
#47268=CARTESIAN_POINT('Ctrl Pts',(-0.273951203132383,-0.950931374872775,
-0.128634819404772));
#47269=CARTESIAN_POINT('Ctrl Pts',(-0.430860211839885,-0.905725604325433,
-0.135202577116414));
#47270=CARTESIAN_POINT('Ctrl Pts',(-0.576352115746697,-0.820857135607116,
-0.141770334828055));
#47271=CARTESIAN_POINT('Ctrl Pts',(-0.692935400633598,-0.706517265211744,
-0.148338092539697));
#47272=CARTESIAN_POINT('Ctrl Pts',(-0.809518685520499,-0.592177394816371,
-0.154905850251338));
#47273=CARTESIAN_POINT('Ctrl Pts',(-0.897193351387491,-0.44836612274394,
-0.161473607962979));
#47274=CARTESIAN_POINT('Ctrl Pts',(-0.94543466694418,-0.292360564284275,
-0.168041365674621));
#47275=CARTESIAN_POINT('Ctrl Pts',(-0.974651086749275,-0.19787881486909,
-0.172019001115677));
#47276=CARTESIAN_POINT('Ctrl Pts',(-0.98940380726374,-0.0989243414783639,
-0.175996636556733));
#47277=CARTESIAN_POINT('Ctrl Pts',(-0.989456987247134,1.47486280241971E-5,
-0.17997427199779));
#47278=CARTESIAN_POINT('Origin',(0.,0.,-0.799));
#47279=CARTESIAN_POINT('',(0.288675134594813,-0.5,-0.799));
#47280=CARTESIAN_POINT('',(-0.288675134594813,-0.5,-0.799));
#47281=CARTESIAN_POINT('',(0.144337567297406,-0.5,-0.799));
#47282=CARTESIAN_POINT('Origin',(0.,0.,-0.799));
#47283=CARTESIAN_POINT('Origin',(0.,0.,-0.799));
#47284=CARTESIAN_POINT('',(-0.577350269189626,2.77555756156289E-16,-0.799));
#47285=CARTESIAN_POINT('',(-0.360843918243516,-0.375,-0.799));
#47286=CARTESIAN_POINT('Origin',(0.,0.,-0.799));
#47287=CARTESIAN_POINT('Origin',(0.,0.,-0.799));
#47288=CARTESIAN_POINT('',(-0.288675134594813,0.5,-0.799));
#47289=CARTESIAN_POINT('',(-0.505181485540923,0.125,-0.799));
#47290=CARTESIAN_POINT('Origin',(0.,0.,-0.799));
#47291=CARTESIAN_POINT('Origin',(0.,0.,-0.799));
#47292=CARTESIAN_POINT('',(0.288675134594813,0.5,-0.799));
#47293=CARTESIAN_POINT('',(-0.144337567297406,0.5,-0.799));
#47294=CARTESIAN_POINT('Origin',(0.,0.,-0.799));
#47295=CARTESIAN_POINT('Origin',(0.,0.,-0.799));
#47296=CARTESIAN_POINT('',(0.577350269189626,0.,-0.799));
#47297=CARTESIAN_POINT('',(0.360843918243516,0.375,-0.799));
#47298=CARTESIAN_POINT('Origin',(0.,0.,-0.799));
#47299=CARTESIAN_POINT('Origin',(0.,0.,-0.799));
#47300=CARTESIAN_POINT('',(0.505181485540923,-0.125,-0.799));
#47301=CARTESIAN_POINT('Origin',(0.,0.,-0.799));
#47302=CARTESIAN_POINT('Origin',(0.,0.,-0.972705080756888));
#47303=CARTESIAN_POINT('',(0.,0.,-1.14641016151378));
#47304=CARTESIAN_POINT('',(-0.575688399926292,-7.05014956275995E-17,-0.8));
#47305=CARTESIAN_POINT('',(-0.288675134594813,-3.53525079574969E-17,-0.972705080756888));
#47306=CARTESIAN_POINT('',(-0.575681140772105,-0.00289101522350376,-0.8));
#47307=CARTESIAN_POINT('Origin',(0.,0.,-0.8));
#47308=CARTESIAN_POINT('Ctrl Pts',(-0.577350269189626,1.38777878078145E-16,
-0.799));
#47309=CARTESIAN_POINT('Ctrl Pts',(-0.576514502127378,-0.00144759101510493,
-0.799502907828364));
#47310=CARTESIAN_POINT('Ctrl Pts',(-0.575681140772105,-0.00289101522350382,
-0.8));
#47311=CARTESIAN_POINT('',(-0.290344263012334,-0.497108984776496,-0.8));
#47312=CARTESIAN_POINT('Ctrl Pts',(-0.290344263012334,-0.497108984776496,
-0.8));
#47313=CARTESIAN_POINT('Ctrl Pts',(-0.289510901657063,-0.498552408984891,
-0.799502907828365));
#47314=CARTESIAN_POINT('Ctrl Pts',(-0.288675134594813,-0.5,-0.799));
#47315=CARTESIAN_POINT('',(-0.285336877759771,-0.5,-0.8));
#47316=CARTESIAN_POINT('Origin',(0.,0.,-0.8));
#47317=CARTESIAN_POINT('Ctrl Pts',(-0.288675134594813,-0.5,-0.799));
#47318=CARTESIAN_POINT('Ctrl Pts',(-0.287003600470267,-0.5,-0.799502907828379));
#47319=CARTESIAN_POINT('Ctrl Pts',(-0.28533687775977,-0.5,-0.8));
#47320=CARTESIAN_POINT('',(0.285336877759771,-0.5,-0.8));
#47321=CARTESIAN_POINT('Ctrl Pts',(0.28533687775977,-0.5,-0.8));
#47322=CARTESIAN_POINT('Ctrl Pts',(0.287003600470239,-0.5,-0.799502907828387));
#47323=CARTESIAN_POINT('Ctrl Pts',(0.288675134594813,-0.5,-0.799));
#47324=CARTESIAN_POINT('',(0.290344263012334,-0.497108984776496,-0.8));
#47325=CARTESIAN_POINT('Origin',(0.,0.,-0.8));
#47326=CARTESIAN_POINT('Ctrl Pts',(0.288675134594813,-0.5,-0.799));
#47327=CARTESIAN_POINT('Ctrl Pts',(0.289510901657071,-0.498552408984877,
-0.79950290782837));
#47328=CARTESIAN_POINT('Ctrl Pts',(0.290344263012334,-0.497108984776496,
-0.8));
#47329=CARTESIAN_POINT('',(0.575681140772105,-0.00289101522350382,-0.8));
#47330=CARTESIAN_POINT('Ctrl Pts',(0.575681140772105,-0.00289101522350412,
-0.8));
#47331=CARTESIAN_POINT('Ctrl Pts',(0.576514502127361,-0.00144759101513511,
-0.799502907828374));
#47332=CARTESIAN_POINT('Ctrl Pts',(0.577350269189626,-3.05311331771918E-16,
-0.799));
#47333=CARTESIAN_POINT('',(0.575681140772105,0.00289101522350384,-0.8));
#47334=CARTESIAN_POINT('Origin',(0.,0.,-0.8));
#47335=CARTESIAN_POINT('Ctrl Pts',(0.577350269189626,4.44089209850062E-16,
-0.799));
#47336=CARTESIAN_POINT('Ctrl Pts',(0.57651450212736,0.00144759101513667,
-0.799502907828375));
#47337=CARTESIAN_POINT('Ctrl Pts',(0.575681140772105,0.00289101522350415,
-0.8));
#47338=CARTESIAN_POINT('',(0.290344263012334,0.497108984776496,-0.8));
#47339=CARTESIAN_POINT('Ctrl Pts',(0.290344263012334,0.497108984776496,
-0.8));
#47340=CARTESIAN_POINT('Ctrl Pts',(0.28951090165707,0.498552408984879,-0.799502907828369));
#47341=CARTESIAN_POINT('Ctrl Pts',(0.288675134594813,0.5,-0.799));
#47342=CARTESIAN_POINT('',(0.28533687775977,0.5,-0.8));
#47343=CARTESIAN_POINT('Origin',(0.,0.,-0.8));
#47344=CARTESIAN_POINT('Ctrl Pts',(0.288675134594813,0.5,-0.799));
#47345=CARTESIAN_POINT('Ctrl Pts',(0.287003600470183,0.5,-0.799502907828404));
#47346=CARTESIAN_POINT('Ctrl Pts',(0.28533687775977,0.5,-0.8));
#47347=CARTESIAN_POINT('',(-0.28533687775977,0.5,-0.8));
#47348=CARTESIAN_POINT('Ctrl Pts',(-0.28533687775977,0.5,-0.8));
#47349=CARTESIAN_POINT('Ctrl Pts',(-0.287003600470227,0.5,-0.799502907828391));
#47350=CARTESIAN_POINT('Ctrl Pts',(-0.288675134594813,0.5,-0.799));
#47351=CARTESIAN_POINT('',(-0.290344263012334,0.497108984776496,-0.8));
#47352=CARTESIAN_POINT('Origin',(0.,0.,-0.8));
#47353=CARTESIAN_POINT('Ctrl Pts',(-0.288675134594813,0.5,-0.799));
#47354=CARTESIAN_POINT('Ctrl Pts',(-0.289510901657074,0.498552408984871,
-0.799502907828372));
#47355=CARTESIAN_POINT('Ctrl Pts',(-0.290344263012334,0.497108984776496,
-0.8));
#47356=CARTESIAN_POINT('',(-0.575681140772105,0.00289101522350423,-0.8));
#47357=CARTESIAN_POINT('Ctrl Pts',(-0.575681140772105,0.00289101522350412,
-0.8));
#47358=CARTESIAN_POINT('Ctrl Pts',(-0.576514502127331,0.00144759101518657,
-0.799502907828392));
#47359=CARTESIAN_POINT('Ctrl Pts',(-0.577350269189626,6.10622663543836E-16,
-0.799));
#47360=CARTESIAN_POINT('Origin',(0.,0.,-0.8));
#47361=CARTESIAN_POINT('Origin',(-0.577350269189626,1.11022302462516E-16,
0.));
#47362=CARTESIAN_POINT('',(-0.288675134594813,0.5,0.));
#47363=CARTESIAN_POINT('',(-0.288675134594813,0.5,0.));
#47364=CARTESIAN_POINT('',(-0.577350269189626,7.07050159149938E-17,0.));
#47365=CARTESIAN_POINT('',(-0.505181485540923,0.125,0.));
#47366=CARTESIAN_POINT('',(-0.577350269189626,7.07050159149938E-17,0.));
#47367=CARTESIAN_POINT('Origin',(-0.577350269189626,1.11022302462516E-16,
0.));
#47368=CARTESIAN_POINT('',(-0.577350269189626,1.11022302462516E-16,-0.8));
#47369=CARTESIAN_POINT('',(-0.577350269189626,7.07050159149938E-17,0.));
#47370=CARTESIAN_POINT('',(-0.288675134594813,0.5,-0.8));
#47371=CARTESIAN_POINT('Origin',(-0.288675134594813,0.5,0.));
#47372=CARTESIAN_POINT('',(0.288675134594813,0.5,0.));
#47373=CARTESIAN_POINT('',(0.288675134594813,0.5,0.));
#47374=CARTESIAN_POINT('',(-0.144337567297406,0.5,0.));
#47375=CARTESIAN_POINT('Origin',(-0.288675134594813,0.5,0.));
#47376=CARTESIAN_POINT('',(0.288675134594813,0.5,-0.8));
#47377=CARTESIAN_POINT('',(0.288675134594813,0.5,-0.8));
#47378=CARTESIAN_POINT('',(0.288675134594813,0.5,0.));
#47379=CARTESIAN_POINT('Origin',(-0.288675134594813,0.5,0.));
#47380=CARTESIAN_POINT('',(-0.288675134594813,0.5,-0.8));
#47381=CARTESIAN_POINT('',(-0.288675134594813,0.5,0.));
#47382=CARTESIAN_POINT('',(0.288675134594813,0.5,-0.8));
#47383=CARTESIAN_POINT('Origin',(-0.288675134594813,-0.5,0.));
#47384=CARTESIAN_POINT('',(-0.288675134594813,-0.5,0.));
#47385=CARTESIAN_POINT('',(-0.360843918243516,-0.375,0.));
#47386=CARTESIAN_POINT('',(-0.288675134594813,-0.5,0.));
#47387=CARTESIAN_POINT('Origin',(-0.288675134594813,-0.5,0.));
#47388=CARTESIAN_POINT('',(-0.288675134594813,-0.5,-0.8));
#47389=CARTESIAN_POINT('',(-0.288675134594813,-0.5,0.));
#47390=CARTESIAN_POINT('',(-0.577350269189626,7.07050159149938E-17,-0.8));
#47391=CARTESIAN_POINT('Origin',(0.288675134594813,0.5,0.));
#47392=CARTESIAN_POINT('',(0.577350269189626,0.,0.));
#47393=CARTESIAN_POINT('',(0.577350269189626,0.,0.));
#47394=CARTESIAN_POINT('',(0.360843918243516,0.375,0.));
#47395=CARTESIAN_POINT('Origin',(0.288675134594813,0.5,0.));
#47396=CARTESIAN_POINT('',(0.577350269189626,0.,-0.8));
#47397=CARTESIAN_POINT('',(0.577350269189626,0.,-0.8));
#47398=CARTESIAN_POINT('',(0.577350269189626,0.,0.));
#47399=CARTESIAN_POINT('Origin',(0.288675134594813,0.5,0.));
#47400=CARTESIAN_POINT('',(0.577350269189626,0.,-0.8));
#47401=CARTESIAN_POINT('Origin',(0.,0.,-0.8));
#47402=CARTESIAN_POINT('',(-0.288675134594813,0.5,-0.8));
#47403=CARTESIAN_POINT('Origin',(0.,0.,-0.8));
#47404=CARTESIAN_POINT('Origin',(0.,0.,-0.8));
#47405=CARTESIAN_POINT('',(0.288675134594813,-0.5,-0.8));
#47406=CARTESIAN_POINT('Origin',(0.,0.,-0.8));
#47407=CARTESIAN_POINT('',(0.288675134594813,-0.5,-0.8));
#47408=CARTESIAN_POINT('',(-0.288675134594813,-0.5,-0.8));
#47409=CARTESIAN_POINT('',(0.288675134594813,-0.5,-0.8));
#47410=CARTESIAN_POINT('Origin',(0.,0.,-0.8));
#47411=CARTESIAN_POINT('',(-0.288675134594813,-0.5,-0.8));
#47412=CARTESIAN_POINT('Origin',(0.,0.,-0.8));
#47413=CARTESIAN_POINT('',(-0.577350269189626,7.07050159149938E-17,-0.8));
#47414=CARTESIAN_POINT('Origin',(0.577350269189626,0.,0.));
#47415=CARTESIAN_POINT('',(0.288675134594813,-0.5,0.));
#47416=CARTESIAN_POINT('',(0.288675134594813,-0.5,0.));
#47417=CARTESIAN_POINT('',(0.505181485540923,-0.125,0.));
#47418=CARTESIAN_POINT('Origin',(0.577350269189626,0.,0.));
#47419=CARTESIAN_POINT('',(0.288675134594813,-0.5,0.));
#47420=CARTESIAN_POINT('Origin',(0.577350269189626,0.,0.));
#47421=CARTESIAN_POINT('Origin',(0.288675134594813,-0.5,0.));
#47422=CARTESIAN_POINT('Origin',(0.288675134594813,-0.5,0.));
#47423=CARTESIAN_POINT('',(0.144337567297406,-0.5,0.));
#47424=CARTESIAN_POINT('Origin',(-0.577350269189626,1.11022302462516E-16,
0.));
#47425=CARTESIAN_POINT('Origin',(-0.288675134594813,-0.5,0.));
#47426=CARTESIAN_POINT('Origin',(0.288675134594813,-0.5,0.));
#47427=CARTESIAN_POINT('Origin',(0.75,0.,-2.));
#47428=CARTESIAN_POINT('',(-0.75,-9.18485099360515E-17,-2.));
#47429=CARTESIAN_POINT('Origin',(0.,0.,-2.));
#47430=CARTESIAN_POINT('Origin',(0.,0.,-1.875));
#47431=CARTESIAN_POINT('',(-0.875,-1.07156594925393E-16,-1.875));
#47432=CARTESIAN_POINT('Origin',(0.,0.,-0.915));
#47433=CARTESIAN_POINT('Origin',(0.,0.,-0.0695250000000001));
#47434=CARTESIAN_POINT('Origin',(0.,0.,-0.04));
#47435=CARTESIAN_POINT('',(-0.92,-1.12667505521556E-16,-6.93889390390723E-18));
#47436=CARTESIAN_POINT('Origin',(0.,0.,0.));
#47437=CARTESIAN_POINT('',(-0.96,-1.17566092718146E-16,-0.04));
#47438=CARTESIAN_POINT('Origin',(0.,0.,0.));
#70730=UNCERTAINTY_MEASURE_WITH_UNIT(LENGTH_MEASURE(0.001),#70758,
'DISTANCE_ACCURACY_VALUE',
'Maximum model space distance between geometric entities at asserted c
onnectivities');
#70740=UNCERTAINTY_MEASURE_WITH_UNIT(LENGTH_MEASURE(0.001),#70758,
'DISTANCE_ACCURACY_VALUE',
'Maximum model space distance between geometric entities at asserted c
onnectivities');
#70747=(
GEOMETRIC_REPRESENTATION_CONTEXT(3)
GLOBAL_UNCERTAINTY_ASSIGNED_CONTEXT((#70730))
GLOBAL_UNIT_ASSIGNED_CONTEXT((#70758,#70760,#70761))
REPRESENTATION_CONTEXT('','3D')
);
#70757=(
GEOMETRIC_REPRESENTATION_CONTEXT(3)
GLOBAL_UNCERTAINTY_ASSIGNED_CONTEXT((#70740))
GLOBAL_UNIT_ASSIGNED_CONTEXT((#70758,#70760,#70761))
REPRESENTATION_CONTEXT('','3D')
);
#70758=(
LENGTH_UNIT()
NAMED_UNIT(*)
SI_UNIT(.CENTI.,.METRE.)
);
#70760=(
NAMED_UNIT(*)
PLANE_ANGLE_UNIT()
SI_UNIT($,.RADIAN.)
);
#70761=(
NAMED_UNIT(*)
SI_UNIT($,.STERADIAN.)
SOLID_ANGLE_UNIT()
);
#70768=SHAPE_DEFINITION_REPRESENTATION(#70784,#70823);
#70784=PRODUCT_DEFINITION_SHAPE('',$,#70840);
#70823=SHAPE_REPRESENTATION('',(#27432),#70747);
#70833=PRODUCT_DEFINITION_CONTEXT('part definition',#70883,'design');
#70840=PRODUCT_DEFINITION('2026-10-19-02-56-05-716',
'15_ISO_4026_M20x20_Lever_Lock_Screw',#70856,#70833);
#70856=PRODUCT_DEFINITION_FORMATION('',$,#70891);
#70883=APPLICATION_CONTEXT(
'Core Data for Automotive Mechanical Design Process');
#70884=PRODUCT_CONTEXT('part definition',#70883,'mechanical');
#70891=PRODUCT('2026-10-19-02-56-05-716',
'15_ISO_4026_M20x20_Lever_Lock_Screw',$,(#70884));
#71048=COLOUR_RGB('Black',0.12,0.14,0.17);
#71049=FILL_AREA_STYLE_COLOUR('',#71048);
#71050=FILL_AREA_STYLE('',(#71049));
#71051=SURFACE_STYLE_FILL_AREA(#71050);
#71052=SURFACE_SIDE_STYLE('',(#71051));
#71053=SURFACE_STYLE_USAGE(.BOTH.,#71052);
#71054=PRESENTATION_STYLE_ASSIGNMENT((#71053));
ENDSEC;
END-ISO-10303-21;
